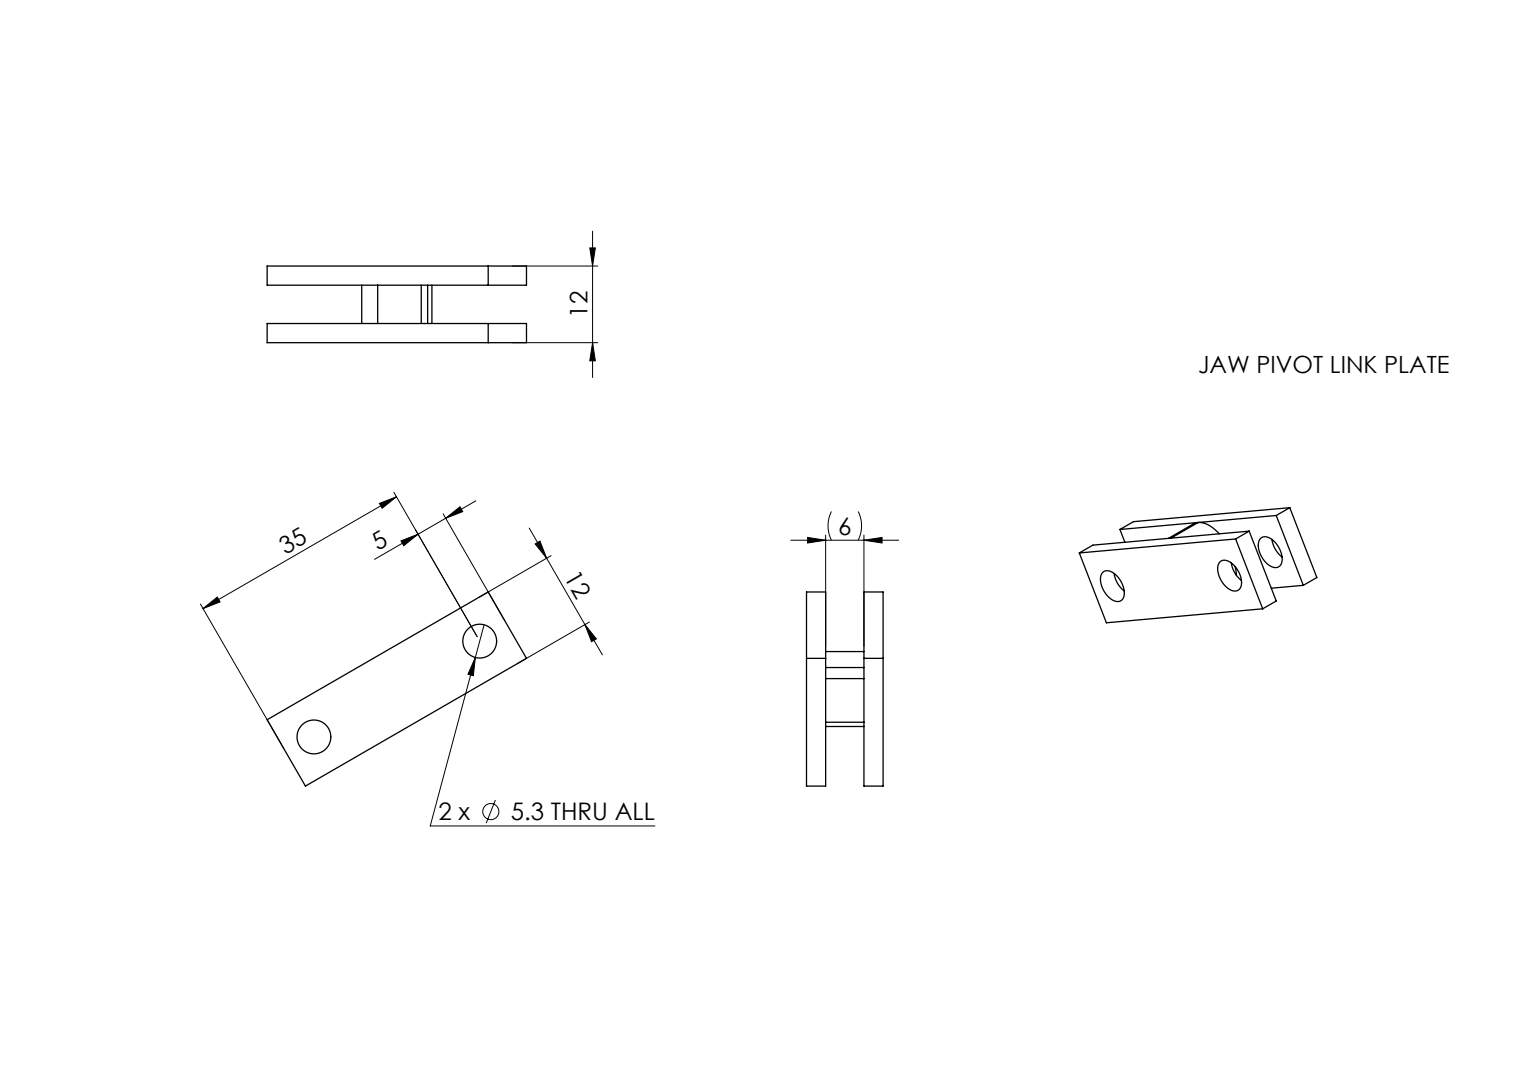
ISO-10303-21;
HEADER;
FILE_DESCRIPTION (('STEP AP214'),
    '1' );
FILE_NAME ('Jaw Pivot Link Plate.step',
    '2026-10-22T13:24:12',
    ( '' ),
    ( '' ),
    'SwSTEP 2.0',
    'SolidWorks 2026',
    '' );
FILE_SCHEMA (( 'AUTOMOTIVE_DESIGN' ));
ENDSEC;

DATA;
#3=AXIS2_PLACEMENT_3D ( 'NONE', #2223, #202, #1998 ) ;
#6=VECTOR ( 'NONE', #2626, 1000.000000000000114 ) ;
#7=VECTOR ( 'NONE', #1963, 1000.000000000000000 ) ;
#9=CARTESIAN_POINT ( 'NONE',  ( -18.00961894323348389, -42.69615242270662492, -3.000000000000000000 ) ) ;
#10=PLANE ( 'NONE',  #689 ) ;
#15=VERTEX_POINT ( 'NONE', #913 ) ;
#16=DIRECTION ( 'NONE',  ( 0.000000000000000000, 0.000000000000000000, -1.000000000000000000 ) ) ;
#19=VECTOR ( 'NONE', #1794, 1000.000000000000000 ) ;
#21=EDGE_CURVE ( 'NONE', #1828, #1252, #472, .T. ) ;
#25=FACE_OUTER_BOUND ( 'NONE', #1470, .T. ) ;
#26=VERTEX_POINT ( 'NONE', #2286 ) ;
#31=FACE_OUTER_BOUND ( 'NONE', #195, .T. ) ;
#32=FACE_OUTER_BOUND ( 'NONE', #973, .T. ) ;
#33=CARTESIAN_POINT ( 'NONE',  ( -32.66987298107778059, -17.30384757729337508, 6.000000000000000000 ) ) ;
#35=DIRECTION ( 'NONE',  ( 1.000000000000000000, 0.000000000000000000, 0.000000000000000000 ) ) ;
#37=CARTESIAN_POINT ( 'NONE',  ( -36.64999999999999147, -25.00000000000000000, 6.000000000000000888 ) ) ;
#38=ADVANCED_FACE ( 'NONE', ( #500, #1172 ), #2089, .T. ) ;
#42=CARTESIAN_POINT ( 'NONE',  ( -43.16025403784440329, -29.13397459621553764, 3.000000000000002220 ) ) ;
#47=EDGE_LOOP ( 'NONE', ( #341, #1054, #52, #1581 ) ) ;
#52=ORIENTED_EDGE ( 'NONE', *, *, #1034, .T. ) ;
#54=AXIS2_PLACEMENT_3D ( 'NONE', #2910, #888, #418 ) ;
#57=ORIENTED_EDGE ( 'NONE', *, *, #910, .F. ) ;
#58=AXIS2_PLACEMENT_3D ( 'NONE', #1165, #883, #1343 ) ;
#60=DIRECTION ( 'NONE',  ( -0.8660254037844401509, -0.4999999999999971689, 1.469576158976821827E-16 ) ) ;
#66=PLANE ( 'NONE',  #2475 ) ;
#68=EDGE_CURVE ( 'NONE', #2151, #2048, #2812, .T. ) ;
#69=LINE ( 'NONE', #303, #372 ) ;
#70=ORIENTED_EDGE ( 'NONE', *, *, #879, .F. ) ;
#72=CARTESIAN_POINT ( 'NONE',  ( -52.65063509461111835, -62.69615242270656807, -3.000000000000000000 ) ) ;
#73=CARTESIAN_POINT ( 'NONE',  ( -43.99038105676666532, -37.69615242270662492, 3.000000000000002665 ) ) ;
#79=FACE_BOUND ( 'NONE', #2327, .T. ) ;
#82=LINE ( 'NONE', #1419, #2817 ) ;
#87=CARTESIAN_POINT ( 'NONE',  ( -59.98076211353318854, -39.99999999999994316, 6.000000000000000888 ) ) ;
#89=LINE ( 'NONE', #2576, #346 ) ;
#92=EDGE_CURVE ( 'NONE', #1675, #1139, #1237, .T. ) ;
#103=VECTOR ( 'NONE', #2064, 1000.000000000000114 ) ;
#105=CARTESIAN_POINT ( 'NONE',  ( -31.00000000000002132, -30.19615242270664268, -3.000000000000000888 ) ) ;
#106=ADVANCED_FACE ( 'NONE', ( #985 ), #566, .F. ) ;
#108=ORIENTED_EDGE ( 'NONE', *, *, #1186, .F. ) ;
#114=LINE ( 'NONE', #1010, #6 ) ;
#116=DIRECTION ( 'NONE',  ( 1.000000000000000000, 0.000000000000000000, 0.000000000000000000 ) ) ;
#117=AXIS2_PLACEMENT_3D ( 'NONE', #1191, #1902, #2801 ) ;
#118=DIRECTION ( 'NONE',  ( 0.000000000000000000, 0.000000000000000000, 1.000000000000000000 ) ) ;
#119=CIRCLE ( 'NONE', #1751, 4.999999999999997335 ) ;
#123=ORIENTED_EDGE ( 'NONE', *, *, #92, .F. ) ;
#124=PRESENTATION_STYLE_ASSIGNMENT (( #2199 ) ) ;
#138=SHAPE_DEFINITION_REPRESENTATION ( #683, #470 ) ;
#139=DIRECTION ( 'NONE',  ( -1.000000000000000000, 0.000000000000000000, 1.272690286469888396E-16 ) ) ;
#140=EDGE_LOOP ( 'NONE', ( #2113, #808, #665, #2884, #381 ) ) ;
#146=ORIENTED_EDGE ( 'NONE', *, *, #1085, .T. ) ;
#148=STYLED_ITEM('',(#2977),#1527);
#150=CIRCLE ( 'NONE', #652, 2.649999999999985700 ) ;
#151=CARTESIAN_POINT ( 'NONE',  ( -31.00000000000002132, -30.19615242270664268, 6.000000000000000000 ) ) ;
#156=CARTESIAN_POINT ( 'NONE',  ( -18.00961894323348389, -42.69615242270662492, 3.000000000000000000 ) ) ;
#161=ADVANCED_FACE ( 'NONE', ( #1024 ), #786, .F. ) ;
#168=DIRECTION ( 'NONE',  ( -0.000000000000000000, -0.000000000000000000, 1.000000000000000000 ) ) ;
#173=CARTESIAN_POINT ( 'NONE',  ( -46.49038105676660848, -33.36602540378440551, -2.999999999999996891 ) ) ;
#178=ADVANCED_FACE ( 'NONE', ( #1439 ), #582, .T. ) ;
#180=CYLINDRICAL_SURFACE ( 'NONE', #659, 2.649999999999985700 ) ;
#181=ORIENTED_EDGE ( 'NONE', *, *, #773, .F. ) ;
#183=FACE_OUTER_BOUND ( 'NONE', #2189, .T. ) ;
#185=CIRCLE ( 'NONE', #2071, 2.649999999999985700 ) ;
#186=DIRECTION ( 'NONE',  ( 1.000000000000000000, 0.000000000000000000, 0.000000000000000000 ) ) ;
#188=EDGE_LOOP ( 'NONE', ( #1239, #2686, #729, #1617 ) ) ;
#189=AXIS2_PLACEMENT_3D ( 'NONE', #2895, #2216, #1972 ) ;
#191=EDGE_CURVE ( 'NONE', #790, #1718, #2828, .T. ) ;
#192=DIRECTION ( 'NONE',  ( -1.076523719386531503E-16, -6.215312591768280423E-17, 1.000000000000000000 ) ) ;
#194=DIRECTION ( 'NONE',  ( 1.000000000000000000, 0.000000000000000000, 0.000000000000000000 ) ) ;
#195=EDGE_LOOP ( 'NONE', ( #2000, #2767, #2469, #1038, #802, #746 ) ) ;
#196=COLOUR_RGB ( '',0.8941176470588234615, 0.8941176470588234615, 0.8941176470588234615 ) ;
#198=LINE ( 'NONE', #2410, #1162 ) ;
#202=DIRECTION ( 'NONE',  ( -0.000000000000000000, -0.000000000000000000, 1.000000000000000000 ) ) ;
#205=DIRECTION ( 'NONE',  ( -1.000000000000000000, 0.000000000000000000, 1.636531581110204284E-16 ) ) ;
#208=EDGE_LOOP ( 'NONE', ( #779, #2624, #1671, #1565 ) ) ;
#210=VECTOR ( 'NONE', #2756, 1000.000000000000000 ) ;
#213=DIRECTION ( 'NONE',  ( -0.000000000000000000, -0.000000000000000000, -1.000000000000000000 ) ) ;
#216=CARTESIAN_POINT ( 'NONE',  ( -31.35000000000001563, -25.00000000000000000, -3.000000000000001332 ) ) ;
#225=DIRECTION ( 'NONE',  ( -0.4999999999999977796, 0.8660254037844399289, 0.000000000000000000 ) ) ;
#229=EDGE_LOOP ( 'NONE', ( #1491, #1391 ) ) ;
#231=CARTESIAN_POINT ( 'NONE',  ( 0.000000000000000000, 0.000000000000000000, 0.000000000000000000 ) ) ;
#234=CARTESIAN_POINT ( 'NONE',  ( -59.98076211353318854, -39.99999999999994316, 3.000000000000000444 ) ) ;
#235=DIRECTION ( 'NONE',  ( -1.000000000000000000, 0.000000000000000000, -0.000000000000000000 ) ) ;
#238=DIRECTION ( 'NONE',  ( -0.000000000000000000, -0.000000000000000000, 1.000000000000000000 ) ) ;
#242=DIRECTION ( 'NONE',  ( -0.000000000000000000, -0.000000000000000000, 1.000000000000000000 ) ) ;
#243=MECHANICAL_DESIGN_GEOMETRIC_PRESENTATION_REPRESENTATION('',(#148),#1694);
#248=AXIS2_PLACEMENT_3D ( 'NONE', #1579, #1566, #1962 ) ;
#251=DIRECTION ( 'NONE',  ( -1.000000000000000000, 0.000000000000000000, 1.272690286469888396E-16 ) ) ;
#261=ORIENTED_EDGE ( 'NONE', *, *, #462, .T. ) ;
#269=ORIENTED_EDGE ( 'NONE', *, *, #725, .T. ) ;
#279=DIRECTION ( 'NONE',  ( 0.8660254037844397068, 0.4999999999999981681, 0.000000000000000000 ) ) ;
#287=CIRCLE ( 'NONE', #2368, 4.999999999999997335 ) ;
#288=ADVANCED_FACE ( 'NONE', ( #385 ), #180, .F. ) ;
#294=VERTEX_POINT ( 'NONE', #1052 ) ;
#296=CARTESIAN_POINT ( 'NONE',  ( -36.99999999999999289, -19.80384757729336087, 3.000000000000004441 ) ) ;
#303=CARTESIAN_POINT ( 'NONE',  ( -31.00000000000002132, -30.19615242270664268, 3.000000000000004441 ) ) ;
#307=ORIENTED_EDGE ( 'NONE', *, *, #364, .F. ) ;
#315=CARTESIAN_POINT ( 'NONE',  ( -57.33076211353320417, -39.99999999999994316, 6.000000000000000000 ) ) ;
#316=ORIENTED_EDGE ( 'NONE', *, *, #1007, .T. ) ;
#317=DIRECTION ( 'NONE',  ( -0.000000000000000000, -0.000000000000000000, -1.000000000000000000 ) ) ;
#319=FACE_OUTER_BOUND ( 'NONE', #1943, .T. ) ;
#321=LINE ( 'NONE', #2557, #1703 ) ;
#324=EDGE_CURVE ( 'NONE', #1945, #2225, #2898, .T. ) ;
#325=ORIENTED_EDGE ( 'NONE', *, *, #21, .F. ) ;
#339=VERTEX_POINT ( 'NONE', #216 ) ;
#340=( NAMED_UNIT ( * ) SI_UNIT ( $, .STERADIAN. ) SOLID_ANGLE_UNIT ( ) );
#341=ORIENTED_EDGE ( 'NONE', *, *, #2493, .T. ) ;
#344=LINE ( 'NONE', #1910, #1067 ) ;
#346=VECTOR ( 'NONE', #1178, 1000.000000000000114 ) ;
#347=DIRECTION ( 'NONE',  ( -0.4999999999999968914, 0.8660254037844404840, 0.000000000000000000 ) ) ;
#349=VERTEX_POINT ( 'NONE', #1259 ) ;
#353=ORIENTED_EDGE ( 'NONE', *, *, #1711, .F. ) ;
#355=EDGE_CURVE ( 'NONE', #1675, #790, #1099, .T. ) ;
#357=CARTESIAN_POINT ( 'NONE',  ( -42.16025403784441039, -30.86602540378440906, -2.999999999999997780 ) ) ;
#363=FILL_AREA_STYLE_COLOUR ( '', #196 ) ;
#364=EDGE_CURVE ( 'NONE', #2326, #862, #2184, .T. ) ;
#366=EDGE_CURVE ( 'NONE', #1139, #1718, #369, .T. ) ;
#369=LINE ( 'NONE', #817, #2570 ) ;
#371=DIRECTION ( 'NONE',  ( -0.000000000000000000, -0.000000000000000000, 1.000000000000000000 ) ) ;
#372=VECTOR ( 'NONE', #1589, 1000.000000000000114 ) ;
#373=EDGE_LOOP ( 'NONE', ( #515, #1717, #2590, #1913 ) ) ;
#376=DIRECTION ( 'NONE',  ( -0.4999999999999981681, 0.8660254037844397068, -0.000000000000000000 ) ) ;
#380=VECTOR ( 'NONE', #213, 1000.000000000000000 ) ;
#381=ORIENTED_EDGE ( 'NONE', *, *, #1328, .F. ) ;
#385=FACE_OUTER_BOUND ( 'NONE', #2331, .T. ) ;
#389=ORIENTED_EDGE ( 'NONE', *, *, #2257, .T. ) ;
#396=ORIENTED_EDGE ( 'NONE', *, *, #1940, .F. ) ;
#398=DIRECTION ( 'NONE',  ( 0.4999999999999977796, -0.8660254037844398178, 0.000000000000000000 ) ) ;
#399=VERTEX_POINT ( 'NONE', #2734 ) ;
#400=ADVANCED_FACE ( 'NONE', ( #439 ), #66, .T. ) ;
#410=CYLINDRICAL_SURFACE ( 'NONE', #3, 2.649999999999985700 ) ;
#412=AXIS2_PLACEMENT_3D ( 'NONE', #1501, #1206, #347 ) ;
#418=DIRECTION ( 'NONE',  ( 1.000000000000000000, 0.000000000000000000, 1.636531581110204284E-16 ) ) ;
#430=DIRECTION ( 'NONE',  ( -0.000000000000000000, -0.000000000000000000, -1.000000000000000000 ) ) ;
#433=DIRECTION ( 'NONE',  ( -1.076523719386531503E-16, -6.215312591768280423E-17, 1.000000000000000000 ) ) ;
#435=CARTESIAN_POINT ( 'NONE',  ( -52.65063509461111835, -62.69615242270656807, 3.000000000000000000 ) ) ;
#438=ORIENTED_EDGE ( 'NONE', *, *, #488, .T. ) ;
#439=FACE_OUTER_BOUND ( 'NONE', #687, .T. ) ;
#445=DIRECTION ( 'NONE',  ( -1.000000000000000000, 0.000000000000000000, 0.000000000000000000 ) ) ;
#446=UNCERTAINTY_MEASURE_WITH_UNIT (LENGTH_MEASURE( 1.000000000000000082E-05 ), #1432, 'distance_accuracy_value', 'NONE');
#455=EDGE_LOOP ( 'NONE', ( #513, #2833, #542, #1258 ) ) ;
#456=DIRECTION ( 'NONE',  ( -0.000000000000000000, -0.000000000000000000, 1.000000000000000000 ) ) ;
#460=FACE_OUTER_BOUND ( 'NONE', #2218, .T. ) ;
#462=EDGE_CURVE ( 'NONE', #349, #2502, #1856, .T. ) ;
#463=CARTESIAN_POINT ( 'NONE',  ( 0.000000000000000000, 0.000000000000000000, 6.000000000000000000 ) ) ;
#467=ORIENTED_EDGE ( 'NONE', *, *, #2602, .T. ) ;
#470=SHAPE_REPRESENTATION ( 'Jaw Pivot Link Plate', ( #2652 ), #836 ) ;
#471=CARTESIAN_POINT ( 'NONE',  ( -51.82050807568884210, -34.13397459621553764, -2.999999999999998224 ) ) ;
#472=LINE ( 'NONE', #1376, #1933 ) ;
#477=DIRECTION ( 'NONE',  ( 0.8660254037844398178, 0.4999999999999977796, 1.243062518353660769E-16 ) ) ;
#481=AXIS2_PLACEMENT_3D ( 'NONE', #2908, #16, #445 ) ;
#482=CIRCLE ( 'NONE', #2858, 4.999999999999997335 ) ;
#486=CARTESIAN_POINT ( 'NONE',  ( -59.98076211353318854, -39.99999999999994316, 6.000000000000000888 ) ) ;
#488=EDGE_CURVE ( 'NONE', #876, #399, #2283, .T. ) ;
#491=EDGE_LOOP ( 'NONE', ( #2013, #70, #820, #269 ) ) ;
#493=CARTESIAN_POINT ( 'NONE',  ( -34.00000000000000000, -25.00000000000000000, 3.000000000000000888 ) ) ;
#496=ORIENTED_EDGE ( 'NONE', *, *, #667, .T. ) ;
#500=FACE_BOUND ( 'NONE', #2907, .T. ) ;
#502=ORIENTED_EDGE ( 'NONE', *, *, #1423, .F. ) ;
#508=ORIENTED_EDGE ( 'NONE', *, *, #725, .F. ) ;
#513=ORIENTED_EDGE ( 'NONE', *, *, #488, .F. ) ;
#515=ORIENTED_EDGE ( 'NONE', *, *, #2863, .F. ) ;
#518=ORIENTED_EDGE ( 'NONE', *, *, #1328, .T. ) ;
#521=EDGE_CURVE ( 'NONE', #1511, #1818, #1561, .T. ) ;
#523=CARTESIAN_POINT ( 'NONE',  ( -49.99038105676663690, -27.30384757729335377, -2.999999999999997335 ) ) ;
#527=ORIENTED_EDGE ( 'NONE', *, *, #1941, .F. ) ;
#534=ORIENTED_EDGE ( 'NONE', *, *, #1800, .T. ) ;
#538=CARTESIAN_POINT ( 'NONE',  ( -41.49038105676660848, -33.36602540378440551, 3.000000000000002665 ) ) ;
#539=ORIENTED_EDGE ( 'NONE', *, *, #2505, .F. ) ;
#540=EDGE_CURVE ( 'NONE', #2636, #730, #82, .T. ) ;
#542=ORIENTED_EDGE ( 'NONE', *, *, #2401, .T. ) ;
#544=CARTESIAN_POINT ( 'NONE',  ( -47.49038105676664401, -31.63397459621555186, 6.000000000000000000 ) ) ;
#545=ORIENTED_EDGE ( 'NONE', *, *, #92, .T. ) ;
#552=AXIS2_PLACEMENT_3D ( 'NONE', #87, #927, #972 ) ;
#553=CARTESIAN_POINT ( 'NONE',  ( -31.00000000000002132, -30.19615242270664268, -6.000000000000000000 ) ) ;
#565=CARTESIAN_POINT ( 'NONE',  ( -39.66025403784451697, -55.19615242270660360, 3.000000000000001776 ) ) ;
#566=PLANE ( 'NONE',  #1377 ) ;
#567=AXIS2_PLACEMENT_3D ( 'NONE', #2486, #2006, #1758 ) ;
#569=AXIS2_PLACEMENT_3D ( 'NONE', #764, #1454, #1672 ) ;
#570=VERTEX_POINT ( 'NONE', #1716 ) ;
#571=ADVANCED_FACE ( 'NONE', ( #2328 ), #967, .F. ) ;
#572=DIRECTION ( 'NONE',  ( -1.076523719386531503E-16, -6.215312591768280423E-17, 1.000000000000000000 ) ) ;
#576=DIRECTION ( 'NONE',  ( -0.000000000000000000, -0.000000000000000000, -1.000000000000000000 ) ) ;
#580=DIRECTION ( 'NONE',  ( 0.8660254037844402619, 0.4999999999999971689, 0.000000000000000000 ) ) ;
#582=CYLINDRICAL_SURFACE ( 'NONE', #117, 4.999999999999997335 ) ;
#584=LINE ( 'NONE', #2391, #2700 ) ;
#585=ORIENTED_EDGE ( 'NONE', *, *, #1155, .T. ) ;
#587=CARTESIAN_POINT ( 'NONE',  ( -34.00000000000000000, -25.00000000000000000, 6.000000000000000000 ) ) ;
#593=AXIS2_PLACEMENT_3D ( 'NONE', #156, #2118, #139 ) ;
#595=PLANE ( 'NONE',  #412 ) ;
#596=CIRCLE ( 'NONE', #2645, 4.999999999999997335 ) ;
#598=ORIENTED_EDGE ( 'NONE', *, *, #1904, .T. ) ;
#600=DIRECTION ( 'NONE',  ( 0.8660254037844401509, 0.4999999999999971689, 1.243062518353660769E-16 ) ) ;
#601=CARTESIAN_POINT ( 'NONE',  ( -62.63076211353317291, -39.99999999999994316, -3.000000000000001332 ) ) ;
#604=DIRECTION ( 'NONE',  ( -1.076523719386531503E-16, -6.215312591768280423E-17, 1.000000000000000000 ) ) ;
#605=VECTOR ( 'NONE', #600, 1000.000000000000114 ) ;
#607=EDGE_CURVE ( 'NONE', #1961, #1828, #1899, .T. ) ;
#610=CLOSED_SHELL ( 'NONE', ( #2194, #161, #1974, #571, #178, #2160, #106, #400, #2246, #2065, #1736, #2154, #1658, #1402, #1315, #699, #2001, #2664, #1386, #38, #2587, #2560, #1195, #1955, #750, #1363, #288, #2829, #1653 ) ) ;
#616=VECTOR ( 'NONE', #2275, 1000.000000000000000 ) ;
#617=CARTESIAN_POINT ( 'NONE',  ( -61.31088913245541505, -47.69615242270656807, 6.000000000000000000 ) ) ;
#620=LINE ( 'NONE', #1802, #616 ) ;
#621=CARTESIAN_POINT ( 'NONE',  ( -31.35000000000001563, -25.00000000000000000, 6.000000000000000000 ) ) ;
#624=EDGE_CURVE ( 'NONE', #2567, #942, #2819, .T. ) ;
#628=CARTESIAN_POINT ( 'NONE',  ( -36.99999999999999289, -19.80384757729336087, 6.000000000000000000 ) ) ;
#629=ORIENTED_EDGE ( 'NONE', *, *, #2417, .T. ) ;
#632=FACE_BOUND ( 'NONE', #1715, .T. ) ;
#633=DIRECTION ( 'NONE',  ( 1.000000000000000000, 0.000000000000000000, 0.000000000000000000 ) ) ;
#635=CYLINDRICAL_SURFACE ( 'NONE', #1883, 4.999999999999997335 ) ;
#638=DIRECTION ( 'NONE',  ( -0.000000000000000000, -0.000000000000000000, -1.000000000000000000 ) ) ;
#642=DIRECTION ( 'NONE',  ( 1.000000000000000000, 0.000000000000000000, 0.000000000000000000 ) ) ;
#647=FACE_OUTER_BOUND ( 'NONE', #1861, .T. ) ;
#649=CARTESIAN_POINT ( 'NONE',  ( -46.49038105676660848, -33.36602540378440551, 3.000000000000002220 ) ) ;
#652=AXIS2_PLACEMENT_3D ( 'NONE', #1004, #572, #1030 ) ;
#654=DIRECTION ( 'NONE',  ( -0.000000000000000000, -0.000000000000000000, 1.000000000000000000 ) ) ;
#657=ORIENTED_EDGE ( 'NONE', *, *, #706, .F. ) ;
#659=AXIS2_PLACEMENT_3D ( 'NONE', #1765, #168, #1063 ) ;
#665=ORIENTED_EDGE ( 'NONE', *, *, #925, .T. ) ;
#667=EDGE_CURVE ( 'NONE', #1818, #1252, #1514, .T. ) ;
#671=EDGE_CURVE ( 'NONE', #1818, #2151, #620, .T. ) ;
#676=DIRECTION ( 'NONE',  ( -0.000000000000000000, -0.000000000000000000, 1.000000000000000000 ) ) ;
#678=LINE ( 'NONE', #1122, #2095 ) ;
#679=EDGE_LOOP ( 'NONE', ( #539, #585, #496, #1836, #2242, #1273, #1936 ) ) ;
#683=PRODUCT_DEFINITION_SHAPE ( 'NONE', 'NONE',  #982 ) ;
#687=EDGE_LOOP ( 'NONE', ( #2861, #960, #108, #2263 ) ) ;
#689=AXIS2_PLACEMENT_3D ( 'NONE', #628, #1053, #1084 ) ;
#691=VECTOR ( 'NONE', #2610, 1000.000000000000000 ) ;
#699=ADVANCED_FACE ( 'NONE', ( #632, #460 ), #2452, .F. ) ;
#702=ORIENTED_EDGE ( 'NONE', *, *, #2333, .F. ) ;
#704=LINE ( 'NONE', #2770, #1369 ) ;
#706=EDGE_CURVE ( 'NONE', #790, #2206, #873, .T. ) ;
#724=DIRECTION ( 'NONE',  ( 0.000000000000000000, 0.000000000000000000, -1.000000000000000000 ) ) ;
#725=EDGE_CURVE ( 'NONE', #2634, #942, #2927, .T. ) ;
#729=ORIENTED_EDGE ( 'NONE', *, *, #1941, .T. ) ;
#730=VERTEX_POINT ( 'NONE', #2210 ) ;
#731=DIRECTION ( 'NONE',  ( -0.000000000000000000, -0.000000000000000000, 1.000000000000000000 ) ) ;
#739=LINE ( 'NONE', #315, #1592 ) ;
#740=CIRCLE ( 'NONE', #2556, 2.649999999999985700 ) ;
#744=AXIS2_PLACEMENT_3D ( 'NONE', #1788, #1569, #633 ) ;
#746=ORIENTED_EDGE ( 'NONE', *, *, #366, .T. ) ;
#747=AXIS2_PLACEMENT_3D ( 'NONE', #1383, #1180, #2773 ) ;
#750=ADVANCED_FACE ( 'NONE', ( #1092 ), #2035, .T. ) ;
#751=CARTESIAN_POINT ( 'NONE',  ( -43.16025403784440329, -29.13397459621553764, -2.999999999999997780 ) ) ;
#757=AXIS2_PLACEMENT_3D ( 'NONE', #1522, #1553, #251 ) ;
#758=CARTESIAN_POINT ( 'NONE',  ( -59.98076211353318854, -39.99999999999994316, -3.000000000000000888 ) ) ;
#761=FACE_OUTER_BOUND ( 'NONE', #2167, .T. ) ;
#764=CARTESIAN_POINT ( 'NONE',  ( -34.00000000000000000, -25.00000000000000000, 3.000000000000000888 ) ) ;
#768=LINE ( 'NONE', #2375, #2747 ) ;
#773=EDGE_CURVE ( 'NONE', #942, #1945, #119, .T. ) ;
#779=ORIENTED_EDGE ( 'NONE', *, *, #671, .F. ) ;
#783=EDGE_CURVE ( 'NONE', #1252, #1204, #482, .T. ) ;
#786=CYLINDRICAL_SURFACE ( 'NONE', #2717, 2.649999999999985700 ) ;
#790=VERTEX_POINT ( 'NONE', #2256 ) ;
#791=( GEOMETRIC_REPRESENTATION_CONTEXT ( 3 ) GLOBAL_UNCERTAINTY_ASSIGNED_CONTEXT ( ( #1365 ) ) GLOBAL_UNIT_ASSIGNED_CONTEXT ( ( #1254, #2877, #2606 ) ) REPRESENTATION_CONTEXT ( 'NONE', 'WORKASPACE' ) );
#799=EDGE_CURVE ( 'NONE', #2318, #570, #1086, .T. ) ;
#802=ORIENTED_EDGE ( 'NONE', *, *, #2239, .F. ) ;
#804=VECTOR ( 'NONE', #946, 1000.000000000000000 ) ;
#805=PRODUCT_CONTEXT ( 'NONE', #2499, 'mechanical' ) ;
#808=ORIENTED_EDGE ( 'NONE', *, *, #1598, .F. ) ;
#810=FACE_OUTER_BOUND ( 'NONE', #2369, .T. ) ;
#816=CARTESIAN_POINT ( 'NONE',  ( -32.66987298107778770, -17.30384757729337508, -3.000000000000000000 ) ) ;
#817=CARTESIAN_POINT ( 'NONE',  ( -52.65063509461111835, -62.69615242270656807, 3.000000000000000000 ) ) ;
#819=CARTESIAN_POINT ( 'NONE',  ( -51.82050807568884210, -34.13397459621553764, 3.000000000000001776 ) ) ;
#820=ORIENTED_EDGE ( 'NONE', *, *, #2257, .F. ) ;
#824=DIRECTION ( 'NONE',  ( 1.272690286469888396E-16, 7.347880794884083251E-17, 1.000000000000000000 ) ) ;
#834=CARTESIAN_POINT ( 'NONE',  ( -67.31088913245538663, -37.30384757729328271, 6.000000000000000000 ) ) ;
#836=( GEOMETRIC_REPRESENTATION_CONTEXT ( 3 ) GLOBAL_UNCERTAINTY_ASSIGNED_CONTEXT ( ( #2258 ) ) GLOBAL_UNIT_ASSIGNED_CONTEXT ( ( #2847, #2142, #340 ) ) REPRESENTATION_CONTEXT ( 'NONE', 'WORKASPACE' ) );
#846=AXIS2_PLACEMENT_3D ( 'NONE', #72, #2552, #2029 ) ;
#850=CARTESIAN_POINT ( 'NONE',  ( -26.66987298107781967, -27.69615242270666045, -6.000000000000000000 ) ) ;
#853=ORIENTED_EDGE ( 'NONE', *, *, #2493, .F. ) ;
#856=CYLINDRICAL_SURFACE ( 'NONE', #248, 2.649999999999985700 ) ;
#862=VERTEX_POINT ( 'NONE', #2094 ) ;
#867=CARTESIAN_POINT ( 'NONE',  ( -34.00000000000000000, -25.00000000000000000, 6.000000000000000888 ) ) ;
#869=DIRECTION ( 'NONE',  ( -0.000000000000000000, -0.000000000000000000, -1.000000000000000000 ) ) ;
#870=DIRECTION ( 'NONE',  ( -1.000000000000000000, 0.000000000000000000, 1.636531581110204284E-16 ) ) ;
#873=LINE ( 'NONE', #2437, #2718 ) ;
#874=FACE_OUTER_BOUND ( 'NONE', #1782, .T. ) ;
#876=VERTEX_POINT ( 'NONE', #1849 ) ;
#877=CARTESIAN_POINT ( 'NONE',  ( -61.31088913245541505, -47.69615242270656807, 6.000000000000000000 ) ) ;
#878=CARTESIAN_POINT ( 'NONE',  ( -61.31088913245541505, -47.69615242270656807, -6.000000000000000000 ) ) ;
#879=EDGE_CURVE ( 'NONE', #2648, #2567, #1381, .T. ) ;
#880=ORIENTED_EDGE ( 'NONE', *, *, #1530, .T. ) ;
#883=DIRECTION ( 'NONE',  ( -0.4999999999999978351, 0.8660254037844399289, 0.000000000000000000 ) ) ;
#886=DIRECTION ( 'NONE',  ( 1.272690286469888396E-16, 7.347880794884083251E-17, 1.000000000000000000 ) ) ;
#888=DIRECTION ( 'NONE',  ( -1.076523719386531503E-16, -6.215312591768280423E-17, 1.000000000000000000 ) ) ;
#903=ORIENTED_EDGE ( 'NONE', *, *, #2472, .T. ) ;
#906=CARTESIAN_POINT ( 'NONE',  ( -36.64999999999999147, -25.00000000000000000, -3.000000000000000444 ) ) ;
#910=EDGE_CURVE ( 'NONE', #2502, #2634, #89, .T. ) ;
#912=DIRECTION ( 'NONE',  ( -1.272690286469888396E-16, -7.347880794884083251E-17, -1.000000000000000000 ) ) ;
#913=CARTESIAN_POINT ( 'NONE',  ( -67.31088913245542926, -37.30384757729331113, -3.000000000000000000 ) ) ;
#914=CARTESIAN_POINT ( 'NONE',  ( -36.64999999999999147, -25.00000000000000000, 3.000000000000001332 ) ) ;
#917=PLANE ( 'NONE',  #2411 ) ;
#918=CARTESIAN_POINT ( 'NONE',  ( -39.66025403784451697, -55.19615242270660360, -2.999999999999998224 ) ) ;
#920=EDGE_CURVE ( 'NONE', #1023, #26, #321, .T. ) ;
#925=EDGE_CURVE ( 'NONE', #294, #2085, #930, .T. ) ;
#927=DIRECTION ( 'NONE',  ( -0.000000000000000000, -0.000000000000000000, 1.000000000000000000 ) ) ;
#930=LINE ( 'NONE', #1442, #804 ) ;
#931=AXIS2_PLACEMENT_3D ( 'NONE', #2480, #2883, #398 ) ;
#938=DIRECTION ( 'NONE',  ( -0.4999999999999981681, 0.8660254037844397068, -0.000000000000000000 ) ) ;
#942=VERTEX_POINT ( 'NONE', #1814 ) ;
#945=ORIENTED_EDGE ( 'NONE', *, *, #2401, .F. ) ;
#946=DIRECTION ( 'NONE',  ( -0.000000000000000000, -0.000000000000000000, -1.000000000000000000 ) ) ;
#948=VECTOR ( 'NONE', #1778, 1000.000000000000227 ) ;
#960=ORIENTED_EDGE ( 'NONE', *, *, #2505, .T. ) ;
#965=FACE_BOUND ( 'NONE', #1338, .T. ) ;
#966=ORIENTED_EDGE ( 'NONE', *, *, #2439, .F. ) ;
#967=CYLINDRICAL_SURFACE ( 'NONE', #2425, 2.649999999999985700 ) ;
#970=DIRECTION ( 'NONE',  ( 1.000000000000000000, -1.387778780781446464E-15, 8.673617379884040402E-17 ) ) ;
#971=EDGE_CURVE ( 'NONE', #1718, #942, #1597, .T. ) ;
#972=DIRECTION ( 'NONE',  ( 1.000000000000000000, 0.000000000000000000, 0.000000000000000000 ) ) ;
#973=EDGE_LOOP ( 'NONE', ( #2546, #534, #1117, #2394 ) ) ;
#977=DIRECTION ( 'NONE',  ( -1.000000000000000000, 0.000000000000000000, -0.000000000000000000 ) ) ;
#979=CIRCLE ( 'NONE', #1730, 2.649999999999985700 ) ;
#980=EDGE_LOOP ( 'NONE', ( #1572, #1607, #2719, #2251, #880, #2436 ) ) ;
#982=PRODUCT_DEFINITION ( 'UNKNOWN', '', #1072, #1803 ) ;
#984=ORIENTED_EDGE ( 'NONE', *, *, #2380, .T. ) ;
#985=FACE_OUTER_BOUND ( 'NONE', #2608, .T. ) ;
#987=CIRCLE ( 'NONE', #1651, 2.649999999999985700 ) ;
#988=DIRECTION ( 'NONE',  ( 1.000000000000000000, 0.000000000000000000, 0.000000000000000000 ) ) ;
#1004=CARTESIAN_POINT ( 'NONE',  ( -59.98076211353318854, -39.99999999999994316, 3.000000000000000444 ) ) ;
#1007=EDGE_CURVE ( 'NONE', #1517, #1797, #1850, .T. ) ;
#1010=CARTESIAN_POINT ( 'NONE',  ( -36.99999999999999289, -19.80384757729336087, 3.000000000000000888 ) ) ;
#1016=LINE ( 'NONE', #2166, #7 ) ;
#1017=ORIENTED_EDGE ( 'NONE', *, *, #1940, .T. ) ;
#1019=ORIENTED_EDGE ( 'NONE', *, *, #706, .T. ) ;
#1021=LINE ( 'NONE', #553, #2649 ) ;
#1023=VERTEX_POINT ( 'NONE', #2245 ) ;
#1024=FACE_OUTER_BOUND ( 'NONE', #1867, .T. ) ;
#1030=DIRECTION ( 'NONE',  ( 1.000000000000000000, 0.000000000000000000, 1.636531581110204284E-16 ) ) ;
#1033=ORIENTED_EDGE ( 'NONE', *, *, #1228, .F. ) ;
#1034=EDGE_CURVE ( 'NONE', #2085, #1023, #2261, .T. ) ;
#1038=ORIENTED_EDGE ( 'NONE', *, *, #521, .T. ) ;
#1042=DIRECTION ( 'NONE',  ( -0.000000000000000000, -0.000000000000000000, 1.000000000000000000 ) ) ;
#1047=DIRECTION ( 'NONE',  ( -1.000000000000000000, 1.387778780781446464E-15, 8.673617379884040402E-17 ) ) ;
#1050=DIRECTION ( 'NONE',  ( -0.4999999999999981681, 0.8660254037844397068, -0.000000000000000000 ) ) ;
#1051=ORIENTED_EDGE ( 'NONE', *, *, #1375, .T. ) ;
#1052=CARTESIAN_POINT ( 'NONE',  ( -61.31088913245547189, -47.69615242270656807, -3.000000000000000000 ) ) ;
#1053=DIRECTION ( 'NONE',  ( -0.4999999999999978351, 0.8660254037844399289, 0.000000000000000000 ) ) ;
#1054=ORIENTED_EDGE ( 'NONE', *, *, #2457, .F. ) ;
#1057=DIRECTION ( 'NONE',  ( -1.272690286469888396E-16, -7.347880794884083251E-17, -1.000000000000000000 ) ) ;
#1063=DIRECTION ( 'NONE',  ( 1.000000000000000000, 0.000000000000000000, 0.000000000000000000 ) ) ;
#1067=VECTOR ( 'NONE', #2157, 1000.000000000000000 ) ;
#1072=PRODUCT_DEFINITION_FORMATION_WITH_SPECIFIED_SOURCE ( 'ANY', '', #1586, .NOT_KNOWN. ) ;
#1084=DIRECTION ( 'NONE',  ( -0.8660254037844398178, -0.4999999999999977796, 0.000000000000000000 ) ) ;
#1085=EDGE_CURVE ( 'NONE', #1775, #2357, #1996, .T. ) ;
#1086=CIRCLE ( 'NONE', #1796, 2.649999999999985700 ) ;
#1089=PLANE ( 'NONE',  #2129 ) ;
#1092=FACE_OUTER_BOUND ( 'NONE', #491, .T. ) ;
#1095=EDGE_CURVE ( 'NONE', #1204, #2567, #678, .T. ) ;
#1098=ORIENTED_EDGE ( 'NONE', *, *, #355, .F. ) ;
#1099=LINE ( 'NONE', #877, #948 ) ;
#1100=DIRECTION ( 'NONE',  ( -0.000000000000000000, -0.000000000000000000, 1.000000000000000000 ) ) ;
#1103=CARTESIAN_POINT ( 'NONE',  ( -31.00000000000002132, -30.19615242270664268, 6.000000000000000000 ) ) ;
#1104=DIRECTION ( 'NONE',  ( -0.4999999999999981681, 0.8660254037844397068, -0.000000000000000000 ) ) ;
#1106=CARTESIAN_POINT ( 'NONE',  ( -49.99038105676663690, -27.30384757729335377, 6.000000000000000000 ) ) ;
#1117=ORIENTED_EDGE ( 'NONE', *, *, #2470, .T. ) ;
#1119=DIRECTION ( 'NONE',  ( 0.8660254037844398178, 0.4999999999999977796, 0.000000000000000000 ) ) ;
#1122=CARTESIAN_POINT ( 'NONE',  ( -31.00000000000008171, -50.19615242270659650, 3.000000000000002220 ) ) ;
#1123=VECTOR ( 'NONE', #676, 1000.000000000000000 ) ;
#1125=ORIENTED_EDGE ( 'NONE', *, *, #2417, .F. ) ;
#1130=AXIS2_PLACEMENT_3D ( 'NONE', #1868, #604, #2862 ) ;
#1131=CARTESIAN_POINT ( 'NONE',  ( -39.66025403784451697, -55.19615242270660360, -2.999999999999998224 ) ) ;
#1139=VERTEX_POINT ( 'NONE', #1368 ) ;
#1143=ORIENTED_EDGE ( 'NONE', *, *, #1904, .F. ) ;
#1144=CARTESIAN_POINT ( 'NONE',  ( -36.64999999999999147, -25.00000000000000000, 6.000000000000000000 ) ) ;
#1151=ORIENTED_EDGE ( 'NONE', *, *, #462, .F. ) ;
#1155=EDGE_CURVE ( 'NONE', #730, #1818, #2672, .T. ) ;
#1161=DIRECTION ( 'NONE',  ( 0.4999999999999981681, -0.8660254037844397068, 0.000000000000000000 ) ) ;
#1162=VECTOR ( 'NONE', #1050, 1000.000000000000000 ) ;
#1163=FACE_OUTER_BOUND ( 'NONE', #47, .T. ) ;
#1165=CARTESIAN_POINT ( 'NONE',  ( -36.99999999999999289, -19.80384757729336087, 6.000000000000000000 ) ) ;
#1168=VECTOR ( 'NONE', #2020, 1000.000000000000000 ) ;
#1169=DIRECTION ( 'NONE',  ( 0.4999999999999977796, -0.8660254037844398178, 0.000000000000000000 ) ) ;
#1171=ORIENTED_EDGE ( 'NONE', *, *, #1530, .F. ) ;
#1172=FACE_OUTER_BOUND ( 'NONE', #980, .T. ) ;
#1174=EDGE_CURVE ( 'NONE', #1517, #862, #2892, .T. ) ;
#1178=DIRECTION ( 'NONE',  ( -0.8660254037844398178, -0.4999999999999977796, 1.469576158976821827E-16 ) ) ;
#1180=DIRECTION ( 'NONE',  ( 1.076523719386531503E-16, 6.215312591768280423E-17, -1.000000000000000000 ) ) ;
#1186=EDGE_CURVE ( 'NONE', #2206, #1884, #2440, .T. ) ;
#1187=DIRECTION ( 'NONE',  ( -1.000000000000000000, 0.000000000000000000, 8.673617379884040402E-17 ) ) ;
#1191=CARTESIAN_POINT ( 'NONE',  ( -46.49038105676660848, -33.36602540378440551, 3.000000000000002220 ) ) ;
#1195=ADVANCED_FACE ( 'NONE', ( #2929 ), #635, .T. ) ;
#1198=DIRECTION ( 'NONE',  ( -0.4999999999999981681, 0.8660254037844397068, 0.000000000000000000 ) ) ;
#1204=VERTEX_POINT ( 'NONE', #2295 ) ;
#1205=DIRECTION ( 'NONE',  ( -0.4999999999999972244, 0.8660254037844402619, 0.000000000000000000 ) ) ;
#1206=DIRECTION ( 'NONE',  ( 0.8660254037844404840, 0.4999999999999968914, -0.000000000000000000 ) ) ;
#1210=PLANE ( 'NONE',  #1213 ) ;
#1213=AXIS2_PLACEMENT_3D ( 'NONE', #2532, #279, #1198 ) ;
#1217=DIRECTION ( 'NONE',  ( 1.000000000000000000, 0.000000000000000000, 1.636531581110204284E-16 ) ) ;
#1221=DIRECTION ( 'NONE',  ( -0.000000000000000000, -0.000000000000000000, 1.000000000000000000 ) ) ;
#1228=EDGE_CURVE ( 'NONE', #2206, #2636, #2111, .T. ) ;
#1236=CARTESIAN_POINT ( 'NONE',  ( -62.63076211353317291, -39.99999999999994316, 6.000000000000000000 ) ) ;
#1237=LINE ( 'NONE', #2146, #2666 ) ;
#1239=ORIENTED_EDGE ( 'NONE', *, *, #1095, .F. ) ;
#1252=VERTEX_POINT ( 'NONE', #538 ) ;
#1254=( LENGTH_UNIT ( ) NAMED_UNIT ( * ) SI_UNIT ( .MILLI., .METRE. ) );
#1256=ORIENTED_EDGE ( 'NONE', *, *, #1085, .F. ) ;
#1258=ORIENTED_EDGE ( 'NONE', *, *, #2481, .F. ) ;
#1259=CARTESIAN_POINT ( 'NONE',  ( -26.66987298107781257, -27.69615242270665689, -3.000000000000000000 ) ) ;
#1262=ORIENTED_EDGE ( 'NONE', *, *, #607, .T. ) ;
#1269=ORIENTED_EDGE ( 'NONE', *, *, #2785, .T. ) ;
#1273=ORIENTED_EDGE ( 'NONE', *, *, #624, .T. ) ;
#1282=ORIENTED_EDGE ( 'NONE', *, *, #1632, .T. ) ;
#1285=SURFACE_STYLE_FILL_AREA ( #2423 ) ;
#1287=ORIENTED_EDGE ( 'NONE', *, *, #2757, .T. ) ;
#1293=LINE ( 'NONE', #834, #2324 ) ;
#1294=ORIENTED_EDGE ( 'NONE', *, *, #1007, .F. ) ;
#1305=VECTOR ( 'NONE', #580, 1000.000000000000000 ) ;
#1308=CARTESIAN_POINT ( 'NONE',  ( -32.66987298107778059, -17.30384757729337508, 6.000000000000000000 ) ) ;
#1309=DIRECTION ( 'NONE',  ( 1.000000000000000000, 0.000000000000000000, 0.000000000000000000 ) ) ;
#1315=ADVANCED_FACE ( 'NONE', ( #79, #965, #1163 ), #2790, .T. ) ;
#1317=AXIS2_PLACEMENT_3D ( 'NONE', #2002, #1331, #205 ) ;
#1320=AXIS2_PLACEMENT_3D ( 'NONE', #1464, #2816, #970 ) ;
#1328=EDGE_CURVE ( 'NONE', #349, #2171, #1988, .T. ) ;
#1330=AXIS2_PLACEMENT_3D ( 'NONE', #2474, #238, #194 ) ;
#1331=DIRECTION ( 'NONE',  ( -1.272690286469888396E-16, -7.347880794884083251E-17, -1.000000000000000000 ) ) ;
#1332=VERTEX_POINT ( 'NONE', #906 ) ;
#1333=DIRECTION ( 'NONE',  ( 1.000000000000000000, 0.000000000000000000, 8.673617379884040402E-17 ) ) ;
#1337=DIRECTION ( 'NONE',  ( -0.8660254037844401509, -0.4999999999999971689, 1.469576158976821827E-16 ) ) ;
#1338=EDGE_LOOP ( 'NONE', ( #1282, #438 ) ) ;
#1343=DIRECTION ( 'NONE',  ( -0.8660254037844398178, -0.4999999999999977796, 0.000000000000000000 ) ) ;
#1347=FACE_BOUND ( 'NONE', #1620, .T. ) ;
#1349=ORIENTED_EDGE ( 'NONE', *, *, #925, .F. ) ;
#1358=VECTOR ( 'NONE', #2234, 1000.000000000000114 ) ;
#1360=DIRECTION ( 'NONE',  ( -1.272690286469888396E-16, -7.347880794884083251E-17, -1.000000000000000000 ) ) ;
#1363=ADVANCED_FACE ( 'NONE', ( #647 ), #1583, .F. ) ;
#1365=UNCERTAINTY_MEASURE_WITH_UNIT (LENGTH_MEASURE( 1.000000000000000082E-05 ), #1254, 'distance_accuracy_value', 'NONE');
#1367=AXIS2_PLACEMENT_3D ( 'NONE', #587, #2842, #1490 ) ;
#1368=CARTESIAN_POINT ( 'NONE',  ( -61.31088913245546479, -47.69615242270656807, 3.000000000000000000 ) ) ;
#1369=VECTOR ( 'NONE', #2541, 1000.000000000000000 ) ;
#1375=EDGE_CURVE ( 'NONE', #2179, #2824, #2270, .T. ) ;
#1376=CARTESIAN_POINT ( 'NONE',  ( -41.49038105676660848, -33.36602540378440551, 3.000000000000002220 ) ) ;
#1377=AXIS2_PLACEMENT_3D ( 'NONE', #1485, #1205, #2836 ) ;
#1381=LINE ( 'NONE', #42, #210 ) ;
#1383=CARTESIAN_POINT ( 'NONE',  ( -47.49038105676664401, -31.63397459621555186, -2.999999999999999112 ) ) ;
#1386=ADVANCED_FACE ( 'NONE', ( #1554, #31 ), #917, .F. ) ;
#1391=ORIENTED_EDGE ( 'NONE', *, *, #799, .T. ) ;
#1402=ADVANCED_FACE ( 'NONE', ( #1347, #1804, #874 ), #1759, .F. ) ;
#1406=LINE ( 'NONE', #2510, #2568 ) ;
#1408=DIRECTION ( 'NONE',  ( 1.000000000000000000, 0.000000000000000000, 1.636531581110204284E-16 ) ) ;
#1411=FACE_OUTER_BOUND ( 'NONE', #188, .T. ) ;
#1413=VECTOR ( 'NONE', #60, 1000.000000000000114 ) ;
#1416=VECTOR ( 'NONE', #1104, 1000.000000000000000 ) ;
#1419=CARTESIAN_POINT ( 'NONE',  ( -26.66987298107781967, -27.69615242270666045, 6.000000000000000000 ) ) ;
#1423=EDGE_CURVE ( 'NONE', #876, #2824, #1773, .T. ) ;
#1432=( LENGTH_UNIT ( ) NAMED_UNIT ( * ) SI_UNIT ( .MILLI., .METRE. ) );
#1433=CARTESIAN_POINT ( 'NONE',  ( -26.66987298107781967, -27.69615242270666045, 6.000000000000000000 ) ) ;
#1439=FACE_OUTER_BOUND ( 'NONE', #373, .T. ) ;
#1441=ORIENTED_EDGE ( 'NONE', *, *, #2863, .T. ) ;
#1442=CARTESIAN_POINT ( 'NONE',  ( -61.31088913245541505, -47.69615242270656807, 6.000000000000000000 ) ) ;
#1448=DIRECTION ( 'NONE',  ( 1.000000000000000000, 0.000000000000000000, 0.000000000000000000 ) ) ;
#1454=DIRECTION ( 'NONE',  ( -1.272690286469888396E-16, -7.347880794884083251E-17, -1.000000000000000000 ) ) ;
#1461=DIRECTION ( 'NONE',  ( 0.8660254037844402619, 0.4999999999999971689, 0.000000000000000000 ) ) ;
#1464=CARTESIAN_POINT ( 'NONE',  ( -46.49038105676664401, -33.36602540378442683, -2.999999999999997335 ) ) ;
#1467=LINE ( 'NONE', #1507, #1647 ) ;
#1468=EDGE_LOOP ( 'NONE', ( #2539, #123, #1942, #2591 ) ) ;
#1470=EDGE_LOOP ( 'NONE', ( #1349, #1287, #2688, #2379 ) ) ;
#1471=VECTOR ( 'NONE', #1337, 1000.000000000000114 ) ;
#1479=EDGE_LOOP ( 'NONE', ( #325, #2585, #2640, #2235 ) ) ;
#1485=CARTESIAN_POINT ( 'NONE',  ( -31.00000000000002132, -30.19615242270664268, 6.000000000000000000 ) ) ;
#1488=ORIENTED_EDGE ( 'NONE', *, *, #2182, .F. ) ;
#1490=DIRECTION ( 'NONE',  ( 1.000000000000000000, 0.000000000000000000, 0.000000000000000000 ) ) ;
#1491=ORIENTED_EDGE ( 'NONE', *, *, #1575, .T. ) ;
#1492=DIRECTION ( 'NONE',  ( -0.000000000000000000, -0.000000000000000000, 1.000000000000000000 ) ) ;
#1497=AXIS2_PLACEMENT_3D ( 'NONE', #758, #2581, #1217 ) ;
#1501=CARTESIAN_POINT ( 'NONE',  ( -32.66987298107778059, -17.30384757729337508, 6.000000000000000000 ) ) ;
#1507=CARTESIAN_POINT ( 'NONE',  ( -52.65063509461111835, -62.69615242270656807, -3.000000000000000000 ) ) ;
#1511=VERTEX_POINT ( 'NONE', #2517 ) ;
#1514=CIRCLE ( 'NONE', #567, 4.999999999999997335 ) ;
#1516=CARTESIAN_POINT ( 'NONE',  ( -43.99038105676666532, -37.69615242270662492, -2.999999999999997335 ) ) ;
#1517=VERTEX_POINT ( 'NONE', #2807 ) ;
#1520=ORIENTED_EDGE ( 'NONE', *, *, #1886, .T. ) ;
#1522=CARTESIAN_POINT ( 'NONE',  ( -18.00961894323348389, -42.69615242270662492, -3.000000000000000000 ) ) ;
#1524=DIRECTION ( 'NONE',  ( -0.000000000000000000, -0.000000000000000000, 1.000000000000000000 ) ) ;
#1526=CARTESIAN_POINT ( 'NONE',  ( -43.16025403784440329, -29.13397459621553764, 3.000000000000002220 ) ) ;
#1527=MANIFOLD_SOLID_BREP ( 'M5 Clearance Hole1', #610 ) ;
#1530=EDGE_CURVE ( 'NONE', #2225, #2634, #1739, .T. ) ;
#1531=ORIENTED_EDGE ( 'NONE', *, *, #2785, .F. ) ;
#1533=LINE ( 'NONE', #1308, #2609 ) ;
#1544=CIRCLE ( 'NONE', #552, 2.649999999999985700 ) ;
#1549=FACE_OUTER_BOUND ( 'NONE', #1687, .T. ) ;
#1550=CARTESIAN_POINT ( 'NONE',  ( -34.00000000000000000, -25.00000000000000000, -3.000000000000000888 ) ) ;
#1553=DIRECTION ( 'NONE',  ( -1.272690286469888396E-16, -7.347880794884083251E-17, -1.000000000000000000 ) ) ;
#1554=FACE_BOUND ( 'NONE', #229, .T. ) ;
#1557=DIRECTION ( 'NONE',  ( 0.000000000000000000, -0.000000000000000000, 1.000000000000000000 ) ) ;
#1559=DIRECTION ( 'NONE',  ( 1.000000000000000000, 0.000000000000000000, 0.000000000000000000 ) ) ;
#1561=CIRCLE ( 'NONE', #1130, 4.999999999999997335 ) ;
#1562=PLANE ( 'NONE',  #931 ) ;
#1565=ORIENTED_EDGE ( 'NONE', *, *, #68, .F. ) ;
#1566=DIRECTION ( 'NONE',  ( -0.000000000000000000, -0.000000000000000000, 1.000000000000000000 ) ) ;
#1567=ORIENTED_EDGE ( 'NONE', *, *, #799, .F. ) ;
#1569=DIRECTION ( 'NONE',  ( -0.000000000000000000, -0.000000000000000000, 1.000000000000000000 ) ) ;
#1572=ORIENTED_EDGE ( 'NONE', *, *, #2757, .F. ) ;
#1575=EDGE_CURVE ( 'NONE', #570, #2318, #150, .T. ) ;
#1579=CARTESIAN_POINT ( 'NONE',  ( -34.00000000000000000, -25.00000000000000000, 6.000000000000000000 ) ) ;
#1581=ORIENTED_EDGE ( 'NONE', *, *, #920, .T. ) ;
#1583=CYLINDRICAL_SURFACE ( 'NONE', #744, 2.649999999999985700 ) ;
#1586=PRODUCT ( 'Jaw Pivot Link Plate', 'Jaw Pivot Link Plate', '', ( #805 ) ) ;
#1587=EDGE_LOOP ( 'NONE', ( #1294, #2579 ) ) ;
#1589=DIRECTION ( 'NONE',  ( 0.8660254037844401509, 0.4999999999999971689, 1.243062518353660769E-16 ) ) ;
#1591=ORIENTED_EDGE ( 'NONE', *, *, #1719, .T. ) ;
#1592=VECTOR ( 'NONE', #1650, 1000.000000000000000 ) ;
#1595=ORIENTED_EDGE ( 'NONE', *, *, #1632, .F. ) ;
#1597=LINE ( 'NONE', #296, #2526 ) ;
#1598=EDGE_CURVE ( 'NONE', #294, #2151, #2822, .T. ) ;
#1602=CARTESIAN_POINT ( 'NONE',  ( 0.000000000000000000, 0.000000000000000000, -6.000000000000000000 ) ) ;
#1606=PLANE ( 'NONE',  #2406 ) ;
#1607=ORIENTED_EDGE ( 'NONE', *, *, #1598, .T. ) ;
#1608=VECTOR ( 'NONE', #317, 1000.000000000000000 ) ;
#1617=ORIENTED_EDGE ( 'NONE', *, *, #879, .T. ) ;
#1620=EDGE_LOOP ( 'NONE', ( #1488, #307 ) ) ;
#1621=DIRECTION ( 'NONE',  ( 0.000000000000000000, -0.000000000000000000, 1.000000000000000000 ) ) ;
#1632=EDGE_CURVE ( 'NONE', #399, #876, #987, .T. ) ;
#1640=LINE ( 'NONE', #1144, #2454 ) ;
#1647=VECTOR ( 'NONE', #376, 1000.000000000000000 ) ;
#1650=DIRECTION ( 'NONE',  ( -0.000000000000000000, -0.000000000000000000, 1.000000000000000000 ) ) ;
#1651=AXIS2_PLACEMENT_3D ( 'NONE', #1769, #456, #186 ) ;
#1653=ADVANCED_FACE ( 'NONE', ( #2494 ), #856, .F. ) ;
#1658=ADVANCED_FACE ( 'NONE', ( #2695 ), #1089, .F. ) ;
#1669=EDGE_CURVE ( 'NONE', #15, #1023, #1293, .T. ) ;
#1671=ORIENTED_EDGE ( 'NONE', *, *, #1800, .F. ) ;
#1672=DIRECTION ( 'NONE',  ( -1.000000000000000000, 0.000000000000000000, 1.636531581110204284E-16 ) ) ;
#1675=VERTEX_POINT ( 'NONE', #617 ) ;
#1676=ORIENTED_EDGE ( 'NONE', *, *, #2692, .F. ) ;
#1677=DIRECTION ( 'NONE',  ( -0.000000000000000000, -0.000000000000000000, 1.000000000000000000 ) ) ;
#1681=LINE ( 'NONE', #1131, #1416 ) ;
#1686=AXIS2_PLACEMENT_3D ( 'NONE', #486, #2389, #1448 ) ;
#1687=EDGE_LOOP ( 'NONE', ( #2193, #57, #2712, #1823, #2155 ) ) ;
#1694=( GEOMETRIC_REPRESENTATION_CONTEXT ( 3 ) GLOBAL_UNCERTAINTY_ASSIGNED_CONTEXT ( ( #446 ) ) GLOBAL_UNIT_ASSIGNED_CONTEXT ( ( #1432, #2339, #2123 ) ) REPRESENTATION_CONTEXT ( 'NONE', 'WORKASPACE' ) );
#1695=LINE ( 'NONE', #2855, #2501 ) ;
#1703=VECTOR ( 'NONE', #2338, 1000.000000000000114 ) ;
#1706=DIRECTION ( 'NONE',  ( -0.4999999999999981681, 0.8660254037844397068, -0.000000000000000000 ) ) ;
#1711=EDGE_CURVE ( 'NONE', #2357, #1775, #1789, .T. ) ;
#1712=CARTESIAN_POINT ( 'NONE',  ( -31.00000000000002132, -30.19615242270664268, -2.999999999999995559 ) ) ;
#1713=CYLINDRICAL_SURFACE ( 'NONE', #1367, 2.649999999999985700 ) ;
#1714=EDGE_CURVE ( 'NONE', #2502, #26, #1533, .T. ) ;
#1715=EDGE_LOOP ( 'NONE', ( #1813, #1591 ) ) ;
#1716=CARTESIAN_POINT ( 'NONE',  ( -57.33076211353320417, -39.99999999999994316, 3.000000000000000888 ) ) ;
#1717=ORIENTED_EDGE ( 'NONE', *, *, #21, .T. ) ;
#1718=VERTEX_POINT ( 'NONE', #2227 ) ;
#1719=EDGE_CURVE ( 'NONE', #1332, #339, #1885, .T. ) ;
#1723=FACE_OUTER_BOUND ( 'NONE', #679, .T. ) ;
#1730=AXIS2_PLACEMENT_3D ( 'NONE', #493, #2353, #2544 ) ;
#1736=ADVANCED_FACE ( 'NONE', ( #1549 ), #2241, .T. ) ;
#1738=MECHANICAL_DESIGN_GEOMETRIC_PRESENTATION_REPRESENTATION('',(#2222),#791);
#1739=CIRCLE ( 'NONE', #747, 4.999999999999997335 ) ;
#1744=ADVANCED_BREP_SHAPE_REPRESENTATION ( '', ( #1527, #2652 ), #836 ) ;
#1751=AXIS2_PLACEMENT_3D ( 'NONE', #2683, #433, #1333 ) ;
#1752=CARTESIAN_POINT ( 'NONE',  ( -57.33076211353320417, -39.99999999999994316, -3.000000000000000444 ) ) ;
#1753=VERTEX_POINT ( 'NONE', #2030 ) ;
#1758=DIRECTION ( 'NONE',  ( -1.000000000000000000, 0.000000000000000000, 8.673617379884040402E-17 ) ) ;
#1759=PLANE ( 'NONE',  #2561 ) ;
#1760=CARTESIAN_POINT ( 'NONE',  ( -32.66987298107778059, -17.30384757729337508, 6.000000000000000000 ) ) ;
#1765=CARTESIAN_POINT ( 'NONE',  ( -59.98076211353318854, -39.99999999999994316, 6.000000000000000000 ) ) ;
#1769=CARTESIAN_POINT ( 'NONE',  ( -59.98076211353318854, -39.99999999999994316, -5.999999999999996447 ) ) ;
#1773=LINE ( 'NONE', #2473, #1123 ) ;
#1775=VERTEX_POINT ( 'NONE', #2302 ) ;
#1778=DIRECTION ( 'NONE',  ( -0.4999999999999977796, 0.8660254037844399289, 0.000000000000000000 ) ) ;
#1779=AXIS2_PLACEMENT_3D ( 'NONE', #544, #118, #988 ) ;
#1781=VECTOR ( 'NONE', #1706, 1000.000000000000000 ) ;
#1782=EDGE_LOOP ( 'NONE', ( #903, #1033, #657, #1098 ) ) ;
#1785=ORIENTED_EDGE ( 'NONE', *, *, #1174, .F. ) ;
#1786=VECTOR ( 'NONE', #1524, 1000.000000000000000 ) ;
#1787=DIRECTION ( 'NONE',  ( -1.000000000000000000, 0.000000000000000000, 8.673617379884040402E-17 ) ) ;
#1788=CARTESIAN_POINT ( 'NONE',  ( -59.98076211353318854, -39.99999999999994316, 6.000000000000000000 ) ) ;
#1789=CIRCLE ( 'NONE', #2226, 2.649999999999985700 ) ;
#1794=DIRECTION ( 'NONE',  ( -0.4999999999999981681, 0.8660254037844397068, -0.000000000000000000 ) ) ;
#1796=AXIS2_PLACEMENT_3D ( 'NONE', #234, #2530, #1408 ) ;
#1797=VERTEX_POINT ( 'NONE', #914 ) ;
#1800=EDGE_CURVE ( 'NONE', #2048, #1511, #704, .T. ) ;
#1802=CARTESIAN_POINT ( 'NONE',  ( -43.99038105676666532, -37.69615242270662492, -2.999999999999999112 ) ) ;
#1803=PRODUCT_DEFINITION_CONTEXT ( 'detailed design', #2654, 'design' ) ;
#1804=FACE_BOUND ( 'NONE', #1859, .T. ) ;
#1805=CARTESIAN_POINT ( 'NONE',  ( -61.31088913245541505, -47.69615242270656807, -6.000000000000000000 ) ) ;
#1808=DIRECTION ( 'NONE',  ( -1.000000000000000000, 0.000000000000000000, 8.673617379884040402E-17 ) ) ;
#1810=VERTEX_POINT ( 'NONE', #2554 ) ;
#1813=ORIENTED_EDGE ( 'NONE', *, *, #2923, .T. ) ;
#1814=CARTESIAN_POINT ( 'NONE',  ( -49.99038105676663690, -27.30384757729335377, 3.000000000000002665 ) ) ;
#1818=VERTEX_POINT ( 'NONE', #73 ) ;
#1820=EDGE_CURVE ( 'NONE', #15, #2634, #1406, .T. ) ;
#1823=ORIENTED_EDGE ( 'NONE', *, *, #920, .F. ) ;
#1828=VERTEX_POINT ( 'NONE', #2317 ) ;
#1836=ORIENTED_EDGE ( 'NONE', *, *, #783, .T. ) ;
#1849=CARTESIAN_POINT ( 'NONE',  ( -62.63076211353317291, -39.99999999999994316, -5.999999999999996447 ) ) ;
#1850=CIRCLE ( 'NONE', #569, 2.649999999999985700 ) ;
#1856=LINE ( 'NONE', #9, #19 ) ;
#1859=EDGE_LOOP ( 'NONE', ( #702, #1143 ) ) ;
#1861=EDGE_LOOP ( 'NONE', ( #502, #1595, #2348, #1051 ) ) ;
#1867=EDGE_LOOP ( 'NONE', ( #353, #1520, #2482, #1125 ) ) ;
#1868=CARTESIAN_POINT ( 'NONE',  ( -46.49038105676664401, -33.36602540378442683, 3.000000000000002665 ) ) ;
#1883=AXIS2_PLACEMENT_3D ( 'NONE', #649, #1557, #2716 ) ;
#1884=VERTEX_POINT ( 'NONE', #2784 ) ;
#1885=CIRCLE ( 'NONE', #1317, 2.649999999999985700 ) ;
#1886=EDGE_CURVE ( 'NONE', #2357, #1332, #1640, .T. ) ;
#1890=DIRECTION ( 'NONE',  ( -0.000000000000000000, -0.000000000000000000, -1.000000000000000000 ) ) ;
#1891=DIRECTION ( 'NONE',  ( 1.000000000000000000, 0.000000000000000000, 0.000000000000000000 ) ) ;
#1899=CIRCLE ( 'NONE', #1939, 4.999999999999997335 ) ;
#1902=DIRECTION ( 'NONE',  ( 0.000000000000000000, -0.000000000000000000, 1.000000000000000000 ) ) ;
#1903=FACE_BOUND ( 'NONE', #1587, .T. ) ;
#1904=EDGE_CURVE ( 'NONE', #1753, #1810, #1544, .T. ) ;
#1910=CARTESIAN_POINT ( 'NONE',  ( -42.16025403784441039, -30.86602540378440906, -2.999999999999997780 ) ) ;
#1913=ORIENTED_EDGE ( 'NONE', *, *, #671, .T. ) ;
#1921=ORIENTED_EDGE ( 'NONE', *, *, #1719, .F. ) ;
#1933=VECTOR ( 'NONE', #1621, 1000.000000000000000 ) ;
#1936=ORIENTED_EDGE ( 'NONE', *, *, #2380, .F. ) ;
#1939=AXIS2_PLACEMENT_3D ( 'NONE', #1952, #2198, #1187 ) ;
#1940=EDGE_CURVE ( 'NONE', #570, #1810, #584, .T. ) ;
#1941=EDGE_CURVE ( 'NONE', #1961, #2648, #1695, .T. ) ;
#1942=ORIENTED_EDGE ( 'NONE', *, *, #355, .T. ) ;
#1943=EDGE_LOOP ( 'NONE', ( #1567, #2762, #598, #396 ) ) ;
#1945=VERTEX_POINT ( 'NONE', #819 ) ;
#1947=DIRECTION ( 'NONE',  ( -0.4999999999999981681, 0.8660254037844397068, -0.000000000000000000 ) ) ;
#1952=CARTESIAN_POINT ( 'NONE',  ( -46.49038105676660848, -33.36602540378440551, -2.999999999999996891 ) ) ;
#1954=ORIENTED_EDGE ( 'NONE', *, *, #324, .F. ) ;
#1955=ADVANCED_FACE ( 'NONE', ( #761 ), #2584, .T. ) ;
#1956=LINE ( 'NONE', #2655, #1358 ) ;
#1961=VERTEX_POINT ( 'NONE', #357 ) ;
#1962=DIRECTION ( 'NONE',  ( 1.000000000000000000, 0.000000000000000000, 0.000000000000000000 ) ) ;
#1963=DIRECTION ( 'NONE',  ( -0.000000000000000000, -0.000000000000000000, 1.000000000000000000 ) ) ;
#1972=DIRECTION ( 'NONE',  ( -1.000000000000000000, 0.000000000000000000, 0.000000000000000000 ) ) ;
#1974=ADVANCED_FACE ( 'NONE', ( #319 ), #2161, .F. ) ;
#1987=DIRECTION ( 'NONE',  ( 0.000000000000000000, 0.000000000000000000, 1.000000000000000000 ) ) ;
#1988=LINE ( 'NONE', #2276, #1168 ) ;
#1990=AXIS2_PLACEMENT_3D ( 'NONE', #2706, #654, #1559 ) ;
#1994=ORIENTED_EDGE ( 'NONE', *, *, #1186, .T. ) ;
#1995=CARTESIAN_POINT ( 'NONE',  ( -51.82050807568884210, -34.13397459621553764, -2.999999999999998224 ) ) ;
#1996=CIRCLE ( 'NONE', #1330, 2.649999999999985700 ) ;
#1998=DIRECTION ( 'NONE',  ( 1.000000000000000000, 0.000000000000000000, 0.000000000000000000 ) ) ;
#2000=ORIENTED_EDGE ( 'NONE', *, *, #971, .T. ) ;
#2001=ADVANCED_FACE ( 'NONE', ( #1903, #1723 ), #2361, .T. ) ;
#2002=CARTESIAN_POINT ( 'NONE',  ( -34.00000000000000000, -25.00000000000000000, -3.000000000000000888 ) ) ;
#2006=DIRECTION ( 'NONE',  ( 1.272690286469888396E-16, 7.347880794884083251E-17, 1.000000000000000000 ) ) ;
#2010=ORIENTED_EDGE ( 'NONE', *, *, #2182, .T. ) ;
#2013=ORIENTED_EDGE ( 'NONE', *, *, #624, .F. ) ;
#2020=DIRECTION ( 'NONE',  ( -0.000000000000000000, -0.000000000000000000, -1.000000000000000000 ) ) ;
#2022=DIRECTION ( 'NONE',  ( -0.4999999999999981681, 0.8660254037844397068, -0.000000000000000000 ) ) ;
#2029=DIRECTION ( 'NONE',  ( 1.000000000000000000, 0.000000000000000000, 1.076523719386531503E-16 ) ) ;
#2030=CARTESIAN_POINT ( 'NONE',  ( -62.63076211353317291, -39.99999999999994316, 6.000000000000000888 ) ) ;
#2031=DIRECTION ( 'NONE',  ( 0.000000000000000000, 0.000000000000000000, 1.000000000000000000 ) ) ;
#2035=CYLINDRICAL_SURFACE ( 'NONE', #481, 4.999999999999997335 ) ;
#2043=DIRECTION ( 'NONE',  ( -0.8660254037844399289, -0.4999999999999978351, 0.000000000000000000 ) ) ;
#2048=VERTEX_POINT ( 'NONE', #2147 ) ;
#2049=CARTESIAN_POINT ( 'NONE',  ( -46.49038105676660848, -33.36602540378440551, 3.000000000000003109 ) ) ;
#2057=CARTESIAN_POINT ( 'NONE',  ( -62.63076211353317291, -39.99999999999994316, 3.000000000000000000 ) ) ;
#2064=DIRECTION ( 'NONE',  ( 0.4999999999999968914, -0.8660254037844404840, 0.000000000000000000 ) ) ;
#2065=ADVANCED_FACE ( 'NONE', ( #2612 ), #595, .T. ) ;
#2067=CARTESIAN_POINT ( 'NONE',  ( -32.66987298107778059, -17.30384757729337508, 6.000000000000000000 ) ) ;
#2071=AXIS2_PLACEMENT_3D ( 'NONE', #867, #1100, #2415 ) ;
#2085=VERTEX_POINT ( 'NONE', #878 ) ;
#2089=PLANE ( 'NONE',  #846 ) ;
#2092=AXIS2_PLACEMENT_3D ( 'NONE', #2152, #824, #1047 ) ;
#2094=CARTESIAN_POINT ( 'NONE',  ( -31.35000000000001563, -25.00000000000000000, 6.000000000000000888 ) ) ;
#2095=VECTOR ( 'NONE', #2022, 1000.000000000000000 ) ;
#2100=ORIENTED_EDGE ( 'NONE', *, *, #1714, .F. ) ;
#2102=CARTESIAN_POINT ( 'NONE',  ( -61.31088913245541505, -47.69615242270656807, 6.000000000000000000 ) ) ;
#2103=ORIENTED_EDGE ( 'NONE', *, *, #1155, .F. ) ;
#2106=ORIENTED_EDGE ( 'NONE', *, *, #1711, .T. ) ;
#2111=LINE ( 'NONE', #33, #103 ) ;
#2113=ORIENTED_EDGE ( 'NONE', *, *, #2692, .T. ) ;
#2114=CARTESIAN_POINT ( 'NONE',  ( -36.64999999999999147, -25.00000000000000000, -5.999999999999996447 ) ) ;
#2118=DIRECTION ( 'NONE',  ( -1.272690286469888396E-16, -7.347880794884083251E-17, -1.000000000000000000 ) ) ;
#2123=( NAMED_UNIT ( * ) SI_UNIT ( $, .STERADIAN. ) SOLID_ANGLE_UNIT ( ) );
#2124=LINE ( 'NONE', #105, #1413 ) ;
#2129=AXIS2_PLACEMENT_3D ( 'NONE', #1103, #2679, #2253 ) ;
#2142=( NAMED_UNIT ( * ) PLANE_ANGLE_UNIT ( ) SI_UNIT ( $, .RADIAN. ) );
#2146=CARTESIAN_POINT ( 'NONE',  ( -61.31088913245541505, -47.69615242270656807, 6.000000000000000000 ) ) ;
#2147=CARTESIAN_POINT ( 'NONE',  ( -50.82050807568884210, -35.86602540378441972, -2.999999999999998224 ) ) ;
#2148=EDGE_LOOP ( 'NONE', ( #1531, #467, #2187, #2010 ) ) ;
#2151=VERTEX_POINT ( 'NONE', #1516 ) ;
#2152=CARTESIAN_POINT ( 'NONE',  ( -47.49038105676660138, -31.63397459621553054, 3.000000000000003109 ) ) ;
#2154=ADVANCED_FACE ( 'NONE', ( #2432 ), #1562, .T. ) ;
#2155=ORIENTED_EDGE ( 'NONE', *, *, #1669, .F. ) ;
#2157=DIRECTION ( 'NONE',  ( 0.000000000000000000, 0.000000000000000000, -1.000000000000000000 ) ) ;
#2160=ADVANCED_FACE ( 'NONE', ( #183 ), #10, .T. ) ;
#2161=CYLINDRICAL_SURFACE ( 'NONE', #2744, 2.649999999999985700 ) ;
#2166=CARTESIAN_POINT ( 'NONE',  ( -36.64999999999999147, -25.00000000000000000, 6.000000000000000000 ) ) ;
#2167=EDGE_LOOP ( 'NONE', ( #1954, #181, #508, #1171 ) ) ;
#2169=DIRECTION ( 'NONE',  ( 1.000000000000000000, 0.000000000000000000, 0.000000000000000000 ) ) ;
#2171=VERTEX_POINT ( 'NONE', #850 ) ;
#2173=LINE ( 'NONE', #151, #1305 ) ;
#2178=CARTESIAN_POINT ( 'NONE',  ( -59.98076211353318854, -39.99999999999994316, 6.000000000000000000 ) ) ;
#2179=VERTEX_POINT ( 'NONE', #1752 ) ;
#2182=EDGE_CURVE ( 'NONE', #862, #2326, #185, .T. ) ;
#2184=CIRCLE ( 'NONE', #1990, 2.649999999999985700 ) ;
#2186=VECTOR ( 'NONE', #1987, 1000.000000000000000 ) ;
#2187=ORIENTED_EDGE ( 'NONE', *, *, #1174, .T. ) ;
#2189=EDGE_LOOP ( 'NONE', ( #984, #2926, #2278, #1019, #1994 ) ) ;
#2193=ORIENTED_EDGE ( 'NONE', *, *, #1820, .T. ) ;
#2194=ADVANCED_FACE ( 'NONE', ( #2446 ), #410, .F. ) ;
#2198=DIRECTION ( 'NONE',  ( -1.272690286469888396E-16, -7.347880794884083251E-17, -1.000000000000000000 ) ) ;
#2199=SURFACE_STYLE_USAGE ( .BOTH. , #2623 ) ;
#2206=VERTEX_POINT ( 'NONE', #2330 ) ;
#2210=CARTESIAN_POINT ( 'NONE',  ( -26.66987298107781257, -27.69615242270665689, 3.000000000000000000 ) ) ;
#2216=DIRECTION ( 'NONE',  ( 0.000000000000000000, 0.000000000000000000, -1.000000000000000000 ) ) ;
#2218=EDGE_LOOP ( 'NONE', ( #2408, #389, #527, #1262, #1441, #1676, #261 ) ) ;
#2222=STYLED_ITEM ( 'NONE', ( #124 ), #1744 ) ;
#2223=CARTESIAN_POINT ( 'NONE',  ( -34.00000000000000000, -25.00000000000000000, 6.000000000000000000 ) ) ;
#2225=VERTEX_POINT ( 'NONE', #471 ) ;
#2226=AXIS2_PLACEMENT_3D ( 'NONE', #2711, #2904, #642 ) ;
#2227=CARTESIAN_POINT ( 'NONE',  ( -67.31088913245542926, -37.30384757729331113, 3.000000000000000000 ) ) ;
#2229=ORIENTED_EDGE ( 'NONE', *, *, #1886, .F. ) ;
#2234=DIRECTION ( 'NONE',  ( 0.4999999999999968914, -0.8660254037844404840, 0.000000000000000000 ) ) ;
#2235=ORIENTED_EDGE ( 'NONE', *, *, #783, .F. ) ;
#2237=VECTOR ( 'NONE', #225, 1000.000000000000227 ) ;
#2239=EDGE_CURVE ( 'NONE', #1139, #1818, #69, .T. ) ;
#2241=PLANE ( 'NONE',  #58 ) ;
#2242=ORIENTED_EDGE ( 'NONE', *, *, #1095, .T. ) ;
#2245=CARTESIAN_POINT ( 'NONE',  ( -67.31088913245538663, -37.30384757729328271, -6.000000000000000000 ) ) ;
#2246=ADVANCED_FACE ( 'NONE', ( #25 ), #1606, .T. ) ;
#2251=ORIENTED_EDGE ( 'NONE', *, *, #2901, .T. ) ;
#2253=DIRECTION ( 'NONE',  ( -0.8660254037844401509, -0.4999999999999971689, 0.000000000000000000 ) ) ;
#2256=CARTESIAN_POINT ( 'NONE',  ( -67.31088913245538663, -37.30384757729328271, 6.000000000000000000 ) ) ;
#2257=EDGE_CURVE ( 'NONE', #2634, #2648, #596, .T. ) ;
#2258=UNCERTAINTY_MEASURE_WITH_UNIT (LENGTH_MEASURE( 1.000000000000000082E-05 ), #2847, 'distance_accuracy_value', 'NONE');
#2259=DIRECTION ( 'NONE',  ( 0.000000000000000000, 0.000000000000000000, -1.000000000000000000 ) ) ;
#2261=LINE ( 'NONE', #1805, #2237 ) ;
#2263=ORIENTED_EDGE ( 'NONE', *, *, #1228, .T. ) ;
#2265=AXIS2_PLACEMENT_3D ( 'NONE', #918, #2808, #1161 ) ;
#2267=CIRCLE ( 'NONE', #1497, 2.649999999999985700 ) ;
#2270=CIRCLE ( 'NONE', #54, 2.649999999999985700 ) ;
#2275=DIRECTION ( 'NONE',  ( -0.000000000000000000, 0.000000000000000000, -1.000000000000000000 ) ) ;
#2276=CARTESIAN_POINT ( 'NONE',  ( -26.66987298107781967, -27.69615242270666045, 6.000000000000000000 ) ) ;
#2278=ORIENTED_EDGE ( 'NONE', *, *, #191, .F. ) ;
#2282=CARTESIAN_POINT ( 'NONE',  ( -59.98076211353318854, -39.99999999999994316, -5.999999999999996447 ) ) ;
#2283=CIRCLE ( 'NONE', #2761, 2.649999999999985700 ) ;
#2286=CARTESIAN_POINT ( 'NONE',  ( -32.66987298107778059, -17.30384757729337508, -6.000000000000000000 ) ) ;
#2295=CARTESIAN_POINT ( 'NONE',  ( -42.16025403784441039, -30.86602540378440906, 3.000000000000002220 ) ) ;
#2302=CARTESIAN_POINT ( 'NONE',  ( -31.35000000000001563, -25.00000000000000000, -5.999999999999996447 ) ) ;
#2317=CARTESIAN_POINT ( 'NONE',  ( -41.49038105676660848, -33.36602540378440551, -2.999999999999997335 ) ) ;
#2318=VERTEX_POINT ( 'NONE', #2057 ) ;
#2324=VECTOR ( 'NONE', #869, 1000.000000000000000 ) ;
#2326=VERTEX_POINT ( 'NONE', #37 ) ;
#2327=EDGE_LOOP ( 'NONE', ( #146, #2106 ) ) ;
#2328=FACE_OUTER_BOUND ( 'NONE', #455, .T. ) ;
#2330=CARTESIAN_POINT ( 'NONE',  ( -32.66987298107778059, -17.30384757729337508, 6.000000000000000000 ) ) ;
#2331=EDGE_LOOP ( 'NONE', ( #966, #2448, #1017, #2443 ) ) ;
#2333=EDGE_CURVE ( 'NONE', #1810, #1753, #2802, .T. ) ;
#2338=DIRECTION ( 'NONE',  ( 0.8660254037844398178, 0.4999999999999977796, 0.000000000000000000 ) ) ;
#2339=( NAMED_UNIT ( * ) PLANE_ANGLE_UNIT ( ) SI_UNIT ( $, .RADIAN. ) );
#2342=ORIENTED_EDGE ( 'NONE', *, *, #1375, .F. ) ;
#2346=CARTESIAN_POINT ( 'NONE',  ( -67.31088913245538663, -37.30384757729328271, 6.000000000000000000 ) ) ;
#2348=ORIENTED_EDGE ( 'NONE', *, *, #2481, .T. ) ;
#2353=DIRECTION ( 'NONE',  ( -1.272690286469888396E-16, -7.347880794884083251E-17, -1.000000000000000000 ) ) ;
#2357=VERTEX_POINT ( 'NONE', #2114 ) ;
#2358=LINE ( 'NONE', #1236, #691 ) ;
#2361=PLANE ( 'NONE',  #593 ) ;
#2368=AXIS2_PLACEMENT_3D ( 'NONE', #173, #1057, #2667 ) ;
#2369=EDGE_LOOP ( 'NONE', ( #2229, #1256, #629, #1921 ) ) ;
#2375=CARTESIAN_POINT ( 'NONE',  ( -31.35000000000001563, -25.00000000000000000, 6.000000000000000000 ) ) ;
#2379=ORIENTED_EDGE ( 'NONE', *, *, #1034, .F. ) ;
#2380=EDGE_CURVE ( 'NONE', #1884, #942, #114, .T. ) ;
#2389=DIRECTION ( 'NONE',  ( -0.000000000000000000, -0.000000000000000000, 1.000000000000000000 ) ) ;
#2391=CARTESIAN_POINT ( 'NONE',  ( -57.33076211353320417, -39.99999999999994316, 6.000000000000000000 ) ) ;
#2394=ORIENTED_EDGE ( 'NONE', *, *, #324, .T. ) ;
#2395=CARTESIAN_POINT ( 'NONE',  ( -59.98076211353318854, -39.99999999999994316, 6.000000000000000000 ) ) ;
#2401=EDGE_CURVE ( 'NONE', #2824, #2179, #2267, .T. ) ;
#2406=AXIS2_PLACEMENT_3D ( 'NONE', #2102, #2043, #1169 ) ;
#2408=ORIENTED_EDGE ( 'NONE', *, *, #910, .T. ) ;
#2410=CARTESIAN_POINT ( 'NONE',  ( -18.00961894323348389, -42.69615242270662492, 3.000000000000000000 ) ) ;
#2411=AXIS2_PLACEMENT_3D ( 'NONE', #435, #192, #2928 ) ;
#2415=DIRECTION ( 'NONE',  ( 1.000000000000000000, 0.000000000000000000, 0.000000000000000000 ) ) ;
#2417=EDGE_CURVE ( 'NONE', #1775, #339, #768, .T. ) ;
#2420=ORIENTED_EDGE ( 'NONE', *, *, #540, .F. ) ;
#2423=FILL_AREA_STYLE ('',( #363 ) ) ;
#2425=AXIS2_PLACEMENT_3D ( 'NONE', #2395, #1492, #2169 ) ;
#2432=FACE_OUTER_BOUND ( 'NONE', #1468, .T. ) ;
#2436=ORIENTED_EDGE ( 'NONE', *, *, #1820, .F. ) ;
#2437=CARTESIAN_POINT ( 'NONE',  ( -36.99999999999999289, -19.80384757729336087, 6.000000000000000000 ) ) ;
#2439=EDGE_CURVE ( 'NONE', #2318, #1753, #2358, .T. ) ;
#2440=LINE ( 'NONE', #1760, #380 ) ;
#2443=ORIENTED_EDGE ( 'NONE', *, *, #2333, .T. ) ;
#2446=FACE_OUTER_BOUND ( 'NONE', #2919, .T. ) ;
#2448=ORIENTED_EDGE ( 'NONE', *, *, #1575, .F. ) ;
#2452=PLANE ( 'NONE',  #757 ) ;
#2454=VECTOR ( 'NONE', #731, 1000.000000000000000 ) ;
#2457=EDGE_CURVE ( 'NONE', #2085, #2171, #1021, .T. ) ;
#2468=EDGE_CURVE ( 'NONE', #1204, #1961, #344, .T. ) ;
#2469=ORIENTED_EDGE ( 'NONE', *, *, #2470, .F. ) ;
#2470=EDGE_CURVE ( 'NONE', #1511, #1945, #2850, .T. ) ;
#2472=EDGE_CURVE ( 'NONE', #1675, #2636, #2173, .T. ) ;
#2473=CARTESIAN_POINT ( 'NONE',  ( -62.63076211353317291, -39.99999999999994316, 6.000000000000000000 ) ) ;
#2474=CARTESIAN_POINT ( 'NONE',  ( -34.00000000000000000, -25.00000000000000000, -5.999999999999996447 ) ) ;
#2475=AXIS2_PLACEMENT_3D ( 'NONE', #2067, #2479, #2503 ) ;
#2479=DIRECTION ( 'NONE',  ( 0.8660254037844404840, 0.4999999999999968914, -0.000000000000000000 ) ) ;
#2480=CARTESIAN_POINT ( 'NONE',  ( -61.31088913245541505, -47.69615242270656807, 6.000000000000000000 ) ) ;
#2481=EDGE_CURVE ( 'NONE', #399, #2179, #739, .T. ) ;
#2482=ORIENTED_EDGE ( 'NONE', *, *, #2923, .F. ) ;
#2486=CARTESIAN_POINT ( 'NONE',  ( -46.49038105676660848, -33.36602540378440551, 3.000000000000003109 ) ) ;
#2493=EDGE_CURVE ( 'NONE', #26, #2171, #1956, .T. ) ;
#2494=FACE_OUTER_BOUND ( 'NONE', #2148, .T. ) ;
#2499=APPLICATION_CONTEXT ( 'automotive_design' ) ;
#2501=VECTOR ( 'NONE', #1947, 1000.000000000000000 ) ;
#2502=VERTEX_POINT ( 'NONE', #816 ) ;
#2503=DIRECTION ( 'NONE',  ( -0.4999999999999968914, 0.8660254037844404840, 0.000000000000000000 ) ) ;
#2505=EDGE_CURVE ( 'NONE', #730, #1884, #198, .T. ) ;
#2509=AXIS2_PLACEMENT_3D ( 'NONE', #1602, #724, #977 ) ;
#2510=CARTESIAN_POINT ( 'NONE',  ( -36.99999999999999289, -19.80384757729336087, -2.999999999999995559 ) ) ;
#2517=CARTESIAN_POINT ( 'NONE',  ( -50.82050807568884210, -35.86602540378441972, 3.000000000000001776 ) ) ;
#2526=VECTOR ( 'NONE', #477, 1000.000000000000114 ) ;
#2528=DIRECTION ( 'NONE',  ( 0.8660254037844398178, 0.4999999999999977796, 1.243062518353660769E-16 ) ) ;
#2530=DIRECTION ( 'NONE',  ( -1.076523719386531503E-16, -6.215312591768280423E-17, 1.000000000000000000 ) ) ;
#2532=CARTESIAN_POINT ( 'NONE',  ( -31.00000000000008171, -50.19615242270659650, 3.000000000000002220 ) ) ;
#2539=ORIENTED_EDGE ( 'NONE', *, *, #366, .F. ) ;
#2541=DIRECTION ( 'NONE',  ( 0.000000000000000000, 0.000000000000000000, 1.000000000000000000 ) ) ;
#2544=DIRECTION ( 'NONE',  ( -1.000000000000000000, 0.000000000000000000, 1.636531581110204284E-16 ) ) ;
#2546=ORIENTED_EDGE ( 'NONE', *, *, #2901, .F. ) ;
#2552=DIRECTION ( 'NONE',  ( -1.076523719386531503E-16, -6.215312591768280423E-17, 1.000000000000000000 ) ) ;
#2554=CARTESIAN_POINT ( 'NONE',  ( -57.33076211353320417, -39.99999999999994316, 6.000000000000000888 ) ) ;
#2556=AXIS2_PLACEMENT_3D ( 'NONE', #1550, #1360, #870 ) ;
#2557=CARTESIAN_POINT ( 'NONE',  ( -36.99999999999999289, -19.80384757729336087, -6.000000000000000000 ) ) ;
#2560=ADVANCED_FACE ( 'NONE', ( #2638 ), #2866, .T. ) ;
#2561=AXIS2_PLACEMENT_3D ( 'NONE', #463, #2259, #235 ) ;
#2567=VERTEX_POINT ( 'NONE', #1526 ) ;
#2568=VECTOR ( 'NONE', #2528, 1000.000000000000114 ) ;
#2569=CARTESIAN_POINT ( 'NONE',  ( -34.00000000000000000, -25.00000000000000000, 6.000000000000000000 ) ) ;
#2570=VECTOR ( 'NONE', #938, 1000.000000000000000 ) ;
#2576=CARTESIAN_POINT ( 'NONE',  ( -36.99999999999999289, -19.80384757729336087, -3.000000000000000888 ) ) ;
#2579=ORIENTED_EDGE ( 'NONE', *, *, #2602, .F. ) ;
#2581=DIRECTION ( 'NONE',  ( -1.076523719386531503E-16, -6.215312591768280423E-17, 1.000000000000000000 ) ) ;
#2584=CYLINDRICAL_SURFACE ( 'NONE', #1779, 4.999999999999997335 ) ;
#2585=ORIENTED_EDGE ( 'NONE', *, *, #607, .F. ) ;
#2587=ADVANCED_FACE ( 'NONE', ( #32 ), #2742, .T. ) ;
#2590=ORIENTED_EDGE ( 'NONE', *, *, #667, .F. ) ;
#2591=ORIENTED_EDGE ( 'NONE', *, *, #191, .T. ) ;
#2602=EDGE_CURVE ( 'NONE', #1797, #1517, #979, .T. ) ;
#2606=( NAMED_UNIT ( * ) SI_UNIT ( $, .STERADIAN. ) SOLID_ANGLE_UNIT ( ) );
#2608=EDGE_LOOP ( 'NONE', ( #2615, #2103, #2420, #2814, #545 ) ) ;
#2609=VECTOR ( 'NONE', #430, 1000.000000000000000 ) ;
#2610=DIRECTION ( 'NONE',  ( -0.000000000000000000, -0.000000000000000000, 1.000000000000000000 ) ) ;
#2612=FACE_OUTER_BOUND ( 'NONE', #2637, .T. ) ;
#2614=VECTOR ( 'NONE', #638, 1000.000000000000000 ) ;
#2615=ORIENTED_EDGE ( 'NONE', *, *, #2239, .T. ) ;
#2623=SURFACE_SIDE_STYLE ('',( #1285 ) ) ;
#2624=ORIENTED_EDGE ( 'NONE', *, *, #521, .F. ) ;
#2626=DIRECTION ( 'NONE',  ( -0.8660254037844398178, -0.4999999999999977796, 1.469576158976821827E-16 ) ) ;
#2634=VERTEX_POINT ( 'NONE', #523 ) ;
#2636=VERTEX_POINT ( 'NONE', #1433 ) ;
#2637=EDGE_LOOP ( 'NONE', ( #1151, #518, #853, #2100 ) ) ;
#2638=FACE_OUTER_BOUND ( 'NONE', #208, .T. ) ;
#2640=ORIENTED_EDGE ( 'NONE', *, *, #2468, .F. ) ;
#2645=AXIS2_PLACEMENT_3D ( 'NONE', #2765, #912, #1808 ) ;
#2648=VERTEX_POINT ( 'NONE', #751 ) ;
#2649=VECTOR ( 'NONE', #1461, 1000.000000000000000 ) ;
#2652=AXIS2_PLACEMENT_3D ( 'NONE', #231, #2031, #1309 ) ;
#2654=APPLICATION_CONTEXT ( 'automotive_design' ) ;
#2655=CARTESIAN_POINT ( 'NONE',  ( -32.66987298107778059, -17.30384757729337508, -6.000000000000000000 ) ) ;
#2664=ADVANCED_FACE ( 'NONE', ( #1411 ), #1210, .T. ) ;
#2666=VECTOR ( 'NONE', #1890, 1000.000000000000000 ) ;
#2667=DIRECTION ( 'NONE',  ( -1.000000000000000000, 0.000000000000000000, 8.673617379884040402E-17 ) ) ;
#2670=SHAPE_REPRESENTATION_RELATIONSHIP ( 'NONE' , 'NONE' ,  #470, #1744 ) ;
#2672=LINE ( 'NONE', #2701, #1471 ) ;
#2679=DIRECTION ( 'NONE',  ( -0.4999999999999972244, 0.8660254037844402619, 0.000000000000000000 ) ) ;
#2683=CARTESIAN_POINT ( 'NONE',  ( -47.49038105676664401, -31.63397459621555186, 3.000000000000002665 ) ) ;
#2686=ORIENTED_EDGE ( 'NONE', *, *, #2468, .T. ) ;
#2688=ORIENTED_EDGE ( 'NONE', *, *, #1669, .T. ) ;
#2692=EDGE_CURVE ( 'NONE', #349, #2151, #2124, .T. ) ;
#2695=FACE_OUTER_BOUND ( 'NONE', #140, .T. ) ;
#2696=ORIENTED_EDGE ( 'NONE', *, *, #364, .T. ) ;
#2700=VECTOR ( 'NONE', #371, 1000.000000000000000 ) ;
#2701=CARTESIAN_POINT ( 'NONE',  ( -31.00000000000002132, -30.19615242270664268, 3.000000000000000888 ) ) ;
#2706=CARTESIAN_POINT ( 'NONE',  ( -34.00000000000000000, -25.00000000000000000, 6.000000000000000888 ) ) ;
#2711=CARTESIAN_POINT ( 'NONE',  ( -34.00000000000000000, -25.00000000000000000, -5.999999999999996447 ) ) ;
#2712=ORIENTED_EDGE ( 'NONE', *, *, #1714, .T. ) ;
#2716=DIRECTION ( 'NONE',  ( 1.000000000000000000, 0.000000000000000000, 0.000000000000000000 ) ) ;
#2717=AXIS2_PLACEMENT_3D ( 'NONE', #2569, #1221, #116 ) ;
#2718=VECTOR ( 'NONE', #1119, 1000.000000000000114 ) ;
#2719=ORIENTED_EDGE ( 'NONE', *, *, #68, .T. ) ;
#2734=CARTESIAN_POINT ( 'NONE',  ( -57.33076211353320417, -39.99999999999994316, -5.999999999999996447 ) ) ;
#2742=PLANE ( 'NONE',  #2265 ) ;
#2744=AXIS2_PLACEMENT_3D ( 'NONE', #2178, #1042, #1891 ) ;
#2747=VECTOR ( 'NONE', #1677, 1000.000000000000000 ) ;
#2756=DIRECTION ( 'NONE',  ( -0.000000000000000000, -0.000000000000000000, 1.000000000000000000 ) ) ;
#2757=EDGE_CURVE ( 'NONE', #294, #15, #1467, .T. ) ;
#2761=AXIS2_PLACEMENT_3D ( 'NONE', #2282, #242, #35 ) ;
#2762=ORIENTED_EDGE ( 'NONE', *, *, #2439, .T. ) ;
#2765=CARTESIAN_POINT ( 'NONE',  ( -47.49038105676660138, -31.63397459621553054, -2.999999999999997335 ) ) ;
#2767=ORIENTED_EDGE ( 'NONE', *, *, #773, .T. ) ;
#2770=CARTESIAN_POINT ( 'NONE',  ( -50.82050807568884210, -35.86602540378441972, 3.000000000000001776 ) ) ;
#2773=DIRECTION ( 'NONE',  ( 1.000000000000000000, 0.000000000000000000, 8.673617379884040402E-17 ) ) ;
#2784=CARTESIAN_POINT ( 'NONE',  ( -32.66987298107778770, -17.30384757729337508, 3.000000000000000000 ) ) ;
#2785=EDGE_CURVE ( 'NONE', #1797, #2326, #1016, .T. ) ;
#2790=PLANE ( 'NONE',  #2509 ) ;
#2801=DIRECTION ( 'NONE',  ( 1.000000000000000000, 0.000000000000000000, 0.000000000000000000 ) ) ;
#2802=CIRCLE ( 'NONE', #1686, 2.649999999999985700 ) ;
#2807=CARTESIAN_POINT ( 'NONE',  ( -31.35000000000001563, -25.00000000000000000, 3.000000000000000444 ) ) ;
#2808=DIRECTION ( 'NONE',  ( -0.8660254037844397068, -0.4999999999999981681, 0.000000000000000000 ) ) ;
#2812=CIRCLE ( 'NONE', #1320, 4.999999999999997335 ) ;
#2814=ORIENTED_EDGE ( 'NONE', *, *, #2472, .F. ) ;
#2816=DIRECTION ( 'NONE',  ( 1.076523719386531503E-16, 6.215312591768280423E-17, -1.000000000000000000 ) ) ;
#2817=VECTOR ( 'NONE', #576, 1000.000000000000000 ) ;
#2819=CIRCLE ( 'NONE', #2092, 4.999999999999997335 ) ;
#2822=LINE ( 'NONE', #1712, #605 ) ;
#2824=VERTEX_POINT ( 'NONE', #601 ) ;
#2828=LINE ( 'NONE', #2346, #1608 ) ;
#2829=ADVANCED_FACE ( 'NONE', ( #810 ), #1713, .F. ) ;
#2833=ORIENTED_EDGE ( 'NONE', *, *, #1423, .T. ) ;
#2836=DIRECTION ( 'NONE',  ( -0.8660254037844401509, -0.4999999999999971689, 0.000000000000000000 ) ) ;
#2842=DIRECTION ( 'NONE',  ( -0.000000000000000000, -0.000000000000000000, 1.000000000000000000 ) ) ;
#2847=( LENGTH_UNIT ( ) NAMED_UNIT ( * ) SI_UNIT ( .MILLI., .METRE. ) );
#2850=LINE ( 'NONE', #565, #1781 ) ;
#2855=CARTESIAN_POINT ( 'NONE',  ( -31.00000000000008171, -50.19615242270659650, -2.999999999999997780 ) ) ;
#2858=AXIS2_PLACEMENT_3D ( 'NONE', #2049, #886, #1787 ) ;
#2861=ORIENTED_EDGE ( 'NONE', *, *, #540, .T. ) ;
#2862=DIRECTION ( 'NONE',  ( 1.000000000000000000, 0.000000000000000000, 8.673617379884040402E-17 ) ) ;
#2863=EDGE_CURVE ( 'NONE', #1828, #2151, #287, .T. ) ;
#2866=CYLINDRICAL_SURFACE ( 'NONE', #189, 4.999999999999997335 ) ;
#2877=( NAMED_UNIT ( * ) PLANE_ANGLE_UNIT ( ) SI_UNIT ( $, .RADIAN. ) );
#2883=DIRECTION ( 'NONE',  ( -0.8660254037844399289, -0.4999999999999978351, 0.000000000000000000 ) ) ;
#2884=ORIENTED_EDGE ( 'NONE', *, *, #2457, .T. ) ;
#2892=LINE ( 'NONE', #621, #1786 ) ;
#2895=CARTESIAN_POINT ( 'NONE',  ( -46.49038105676664401, -33.36602540378442683, -2.999999999999998224 ) ) ;
#2898=LINE ( 'NONE', #1995, #2614 ) ;
#2901=EDGE_CURVE ( 'NONE', #2048, #2225, #1681, .T. ) ;
#2904=DIRECTION ( 'NONE',  ( -0.000000000000000000, -0.000000000000000000, 1.000000000000000000 ) ) ;
#2907=EDGE_LOOP ( 'NONE', ( #2342, #945 ) ) ;
#2908=CARTESIAN_POINT ( 'NONE',  ( -47.49038105676660138, -31.63397459621553054, 6.000000000000000000 ) ) ;
#2910=CARTESIAN_POINT ( 'NONE',  ( -59.98076211353318854, -39.99999999999994316, -3.000000000000000888 ) ) ;
#2919=EDGE_LOOP ( 'NONE', ( #316, #1269, #2696, #1785 ) ) ;
#2923=EDGE_CURVE ( 'NONE', #339, #1332, #740, .T. ) ;
#2926=ORIENTED_EDGE ( 'NONE', *, *, #971, .F. ) ;
#2927=LINE ( 'NONE', #1106, #2186 ) ;
#2928=DIRECTION ( 'NONE',  ( 1.000000000000000000, 0.000000000000000000, 1.076523719386531503E-16 ) ) ;
#2929=FACE_OUTER_BOUND ( 'NONE', #1479, .T. ) ;
#2971=COLOUR_RGB('Off White',0.89,0.88,0.83);
#2972=FILL_AREA_STYLE_COLOUR('',#2971);
#2973=FILL_AREA_STYLE('',(#2972));
#2974=SURFACE_STYLE_FILL_AREA(#2973);
#2975=SURFACE_SIDE_STYLE('',(#2974));
#2976=SURFACE_STYLE_USAGE(.BOTH.,#2975);
#2977=PRESENTATION_STYLE_ASSIGNMENT((#2976));
ENDSEC;
END-ISO-10303-21;
